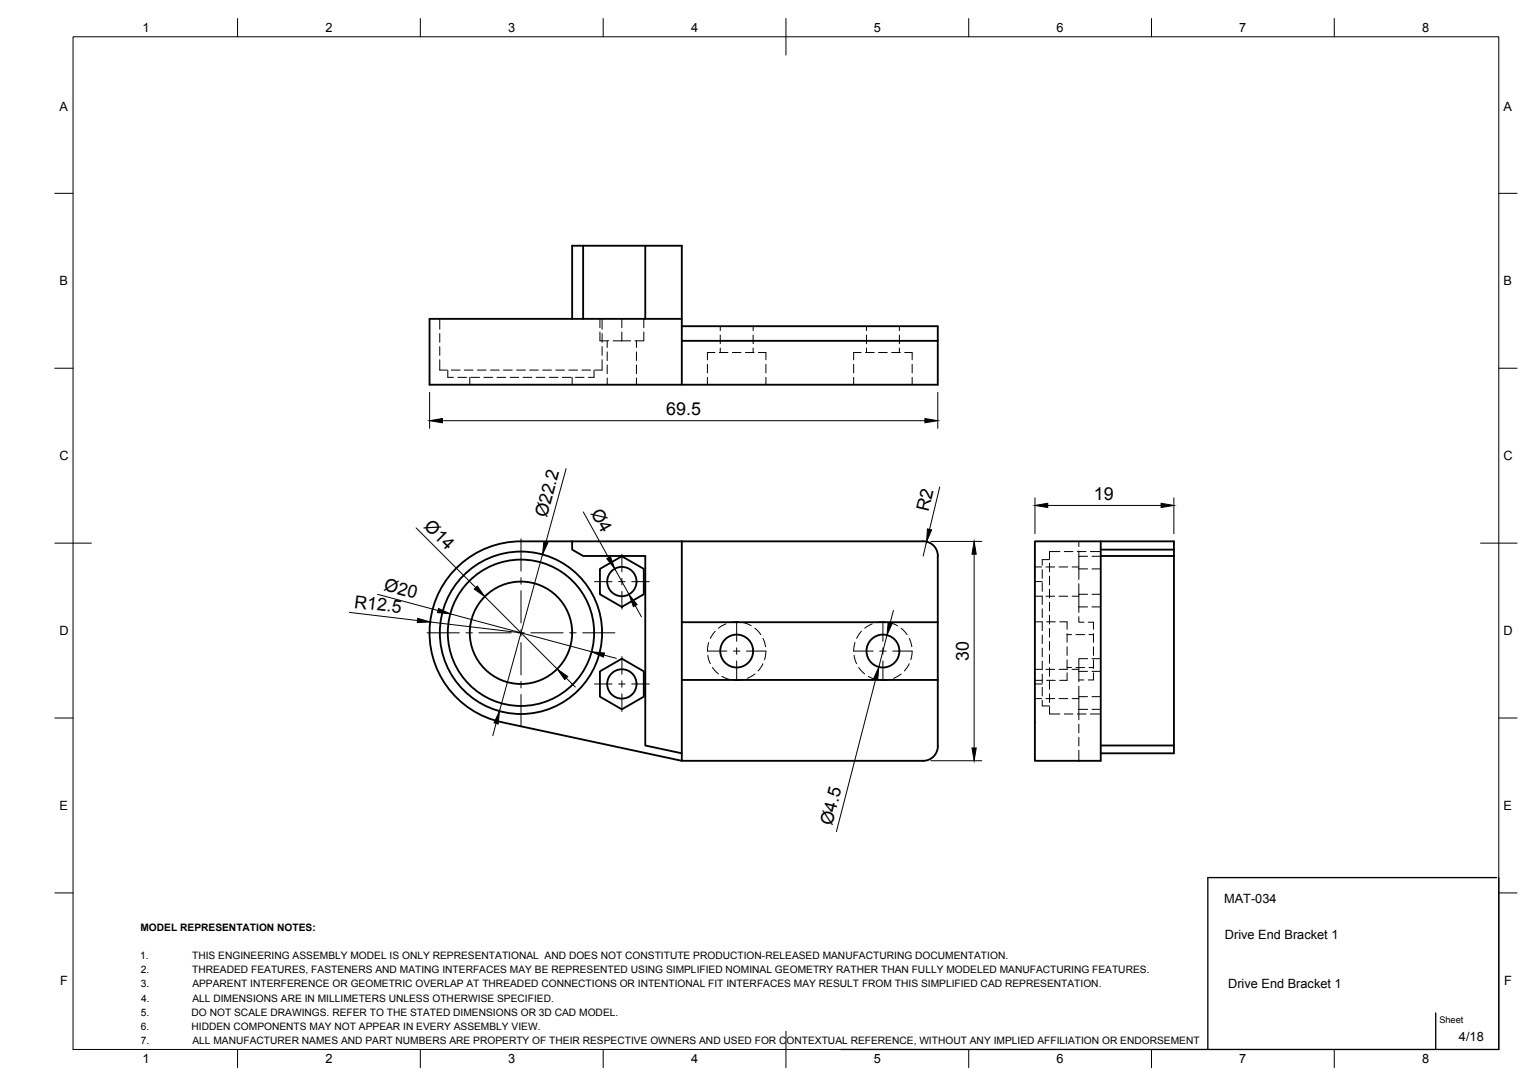
ISO-10303-21;
HEADER;
/* Generated by software containing ST-Developer
 * from STEP Tools, Inc. (www.steptools.com) 
 */

FILE_DESCRIPTION(
/* description */ ('STEP AP214'),
/* implementation_level */ '2;1');

FILE_NAME(
/* name */ 'Drive End Bracket 1.step',
/* time_stamp */ '2026-11-14T09:24:36-08:00',
/* author */ (''),
/* organization */ (''),
/* preprocessor_version */ 'ST-DEVELOPER v20.2',
/* originating_system */ 'Autodesk Translation Framework v15.17.0.0',
/* authorisation */ '');

FILE_SCHEMA (('AUTOMOTIVE_DESIGN { 1 0 10303 214 3 1 1 }'));
ENDSEC;

DATA;
#10=MECHANICAL_DESIGN_GEOMETRIC_PRESENTATION_REPRESENTATION('',(#203),#18867);
#171=SHAPE_REPRESENTATION_RELATIONSHIP('SRR','None',#18935,#187);
#187=ADVANCED_BREP_SHAPE_REPRESENTATION('',(#227),#18851);
#203=STYLED_ITEM('',(#19024),#227);
#227=MANIFOLD_SOLID_BREP('Body1',#10958);
#251=FACE_BOUND('',#1334,.T.);
#252=FACE_BOUND('',#1335,.T.);
#253=FACE_BOUND('',#1336,.T.);
#254=FACE_BOUND('',#1343,.T.);
#255=FACE_BOUND('',#1344,.T.);
#256=FACE_BOUND('',#1345,.T.);
#257=FACE_BOUND('',#1346,.T.);
#258=FACE_BOUND('',#1347,.T.);
#259=FACE_BOUND('',#1349,.T.);
#260=FACE_BOUND('',#1351,.T.);
#261=FACE_BOUND('',#1358,.T.);
#262=FACE_BOUND('',#1360,.T.);
#263=FACE_BOUND('',#1368,.T.);
#264=FACE_BOUND('',#1376,.T.);
#265=FACE_BOUND('',#1381,.T.);
#266=FACE_BOUND('',#1382,.T.);
#381=PLANE('',#11188);
#382=PLANE('',#11189);
#383=PLANE('',#11191);
#384=PLANE('',#11193);
#385=PLANE('',#11195);
#386=PLANE('',#11198);
#387=PLANE('',#11199);
#388=PLANE('',#11200);
#389=PLANE('',#11201);
#390=PLANE('',#11204);
#391=PLANE('',#11205);
#392=PLANE('',#11206);
#393=PLANE('',#11207);
#394=PLANE('',#11208);
#395=PLANE('',#11211);
#396=PLANE('',#11212);
#397=PLANE('',#11213);
#398=PLANE('',#11214);
#399=PLANE('',#11215);
#400=PLANE('',#11216);
#401=PLANE('',#11217);
#402=PLANE('',#11218);
#403=PLANE('',#11219);
#404=PLANE('',#11220);
#405=PLANE('',#11221);
#406=PLANE('',#11222);
#407=PLANE('',#11223);
#408=PLANE('',#11224);
#409=PLANE('',#11225);
#410=PLANE('',#11226);
#411=PLANE('',#11227);
#412=PLANE('',#11228);
#413=PLANE('',#11229);
#414=PLANE('',#11230);
#415=PLANE('',#11231);
#416=PLANE('',#11232);
#725=FACE_OUTER_BOUND('',#1321,.T.);
#726=FACE_OUTER_BOUND('',#1322,.T.);
#727=FACE_OUTER_BOUND('',#1323,.T.);
#728=FACE_OUTER_BOUND('',#1324,.T.);
#729=FACE_OUTER_BOUND('',#1325,.T.);
#730=FACE_OUTER_BOUND('',#1326,.T.);
#731=FACE_OUTER_BOUND('',#1327,.T.);
#732=FACE_OUTER_BOUND('',#1328,.T.);
#733=FACE_OUTER_BOUND('',#1329,.T.);
#734=FACE_OUTER_BOUND('',#1330,.T.);
#735=FACE_OUTER_BOUND('',#1331,.T.);
#736=FACE_OUTER_BOUND('',#1332,.T.);
#737=FACE_OUTER_BOUND('',#1333,.T.);
#738=FACE_OUTER_BOUND('',#1337,.T.);
#739=FACE_OUTER_BOUND('',#1338,.T.);
#740=FACE_OUTER_BOUND('',#1339,.T.);
#741=FACE_OUTER_BOUND('',#1340,.T.);
#742=FACE_OUTER_BOUND('',#1341,.T.);
#743=FACE_OUTER_BOUND('',#1342,.T.);
#744=FACE_OUTER_BOUND('',#1348,.T.);
#745=FACE_OUTER_BOUND('',#1350,.T.);
#746=FACE_OUTER_BOUND('',#1352,.T.);
#747=FACE_OUTER_BOUND('',#1353,.T.);
#748=FACE_OUTER_BOUND('',#1354,.T.);
#749=FACE_OUTER_BOUND('',#1355,.T.);
#750=FACE_OUTER_BOUND('',#1356,.T.);
#751=FACE_OUTER_BOUND('',#1357,.T.);
#752=FACE_OUTER_BOUND('',#1359,.T.);
#753=FACE_OUTER_BOUND('',#1361,.T.);
#754=FACE_OUTER_BOUND('',#1362,.T.);
#755=FACE_OUTER_BOUND('',#1363,.T.);
#756=FACE_OUTER_BOUND('',#1364,.T.);
#757=FACE_OUTER_BOUND('',#1365,.T.);
#758=FACE_OUTER_BOUND('',#1366,.T.);
#759=FACE_OUTER_BOUND('',#1367,.T.);
#760=FACE_OUTER_BOUND('',#1369,.T.);
#761=FACE_OUTER_BOUND('',#1370,.T.);
#762=FACE_OUTER_BOUND('',#1371,.T.);
#763=FACE_OUTER_BOUND('',#1372,.T.);
#764=FACE_OUTER_BOUND('',#1373,.T.);
#765=FACE_OUTER_BOUND('',#1374,.T.);
#766=FACE_OUTER_BOUND('',#1375,.T.);
#767=FACE_OUTER_BOUND('',#1377,.T.);
#768=FACE_OUTER_BOUND('',#1378,.T.);
#769=FACE_OUTER_BOUND('',#1379,.T.);
#770=FACE_OUTER_BOUND('',#1380,.T.);
#771=FACE_OUTER_BOUND('',#1383,.T.);
#772=FACE_OUTER_BOUND('',#1384,.T.);
#1321=EDGE_LOOP('',(#7108,#7109,#7110,#7111));
#1322=EDGE_LOOP('',(#7112,#7113,#7114,#7115));
#1323=EDGE_LOOP('',(#7116,#7117,#7118,#7119));
#1324=EDGE_LOOP('',(#7120,#7121,#7122,#7123));
#1325=EDGE_LOOP('',(#7124,#7125,#7126,#7127));
#1326=EDGE_LOOP('',(#7128,#7129,#7130,#7131));
#1327=EDGE_LOOP('',(#7132,#7133,#7134,#7135));
#1328=EDGE_LOOP('',(#7136,#7137,#7138,#7139));
#1329=EDGE_LOOP('',(#7140,#7141,#7142,#7143));
#1330=EDGE_LOOP('',(#7144,#7145,#7146,#7147,#7148,#7149,#7150,#7151,#7152,
#7153));
#1331=EDGE_LOOP('',(#7154,#7155,#7156,#7157,#7158));
#1332=EDGE_LOOP('',(#7159,#7160,#7161,#7162,#7163));
#1333=EDGE_LOOP('',(#7164,#7165,#7166,#7167,#7168,#7169,#7170,#7171,#7172));
#1334=EDGE_LOOP('',(#7173,#7174,#7175,#7176,#7177,#7178));
#1335=EDGE_LOOP('',(#7179,#7180,#7181,#7182,#7183,#7184));
#1336=EDGE_LOOP('',(#7185));
#1337=EDGE_LOOP('',(#7186,#7187,#7188,#7189,#7190));
#1338=EDGE_LOOP('',(#7191,#7192,#7193,#7194));
#1339=EDGE_LOOP('',(#7195,#7196,#7197,#7198,#7199,#7200,#7201,#7202));
#1340=EDGE_LOOP('',(#7203,#7204,#7205,#7206,#7207,#7208,#7209,#7210));
#1341=EDGE_LOOP('',(#7211,#7212,#7213,#7214));
#1342=EDGE_LOOP('',(#7215,#7216,#7217,#7218,#7219,#7220,#7221));
#1343=EDGE_LOOP('',(#7222));
#1344=EDGE_LOOP('',(#7223));
#1345=EDGE_LOOP('',(#7224));
#1346=EDGE_LOOP('',(#7225));
#1347=EDGE_LOOP('',(#7226));
#1348=EDGE_LOOP('',(#7227));
#1349=EDGE_LOOP('',(#7228));
#1350=EDGE_LOOP('',(#7229));
#1351=EDGE_LOOP('',(#7230));
#1352=EDGE_LOOP('',(#7231,#7232,#7233,#7234));
#1353=EDGE_LOOP('',(#7235,#7236,#7237,#7238));
#1354=EDGE_LOOP('',(#7239,#7240,#7241,#7242,#7243,#7244,#7245));
#1355=EDGE_LOOP('',(#7246,#7247,#7248,#7249));
#1356=EDGE_LOOP('',(#7250,#7251,#7252,#7253));
#1357=EDGE_LOOP('',(#7254));
#1358=EDGE_LOOP('',(#7255));
#1359=EDGE_LOOP('',(#7256));
#1360=EDGE_LOOP('',(#7257));
#1361=EDGE_LOOP('',(#7258,#7259,#7260,#7261));
#1362=EDGE_LOOP('',(#7262,#7263,#7264,#7265));
#1363=EDGE_LOOP('',(#7266,#7267,#7268,#7269));
#1364=EDGE_LOOP('',(#7270,#7271,#7272,#7273));
#1365=EDGE_LOOP('',(#7274,#7275,#7276,#7277));
#1366=EDGE_LOOP('',(#7278,#7279,#7280,#7281));
#1367=EDGE_LOOP('',(#7282,#7283,#7284,#7285,#7286,#7287));
#1368=EDGE_LOOP('',(#7288));
#1369=EDGE_LOOP('',(#7289,#7290,#7291,#7292));
#1370=EDGE_LOOP('',(#7293,#7294,#7295,#7296));
#1371=EDGE_LOOP('',(#7297,#7298,#7299,#7300));
#1372=EDGE_LOOP('',(#7301,#7302,#7303,#7304));
#1373=EDGE_LOOP('',(#7305,#7306,#7307,#7308));
#1374=EDGE_LOOP('',(#7309,#7310,#7311,#7312));
#1375=EDGE_LOOP('',(#7313,#7314,#7315,#7316,#7317,#7318));
#1376=EDGE_LOOP('',(#7319));
#1377=EDGE_LOOP('',(#7320,#7321,#7322,#7323));
#1378=EDGE_LOOP('',(#7324,#7325,#7326,#7327));
#1379=EDGE_LOOP('',(#7328,#7329,#7330,#7331));
#1380=EDGE_LOOP('',(#7332,#7333,#7334,#7335));
#1381=EDGE_LOOP('',(#7336));
#1382=EDGE_LOOP('',(#7337));
#1383=EDGE_LOOP('',(#7338,#7339,#7340,#7341));
#1384=EDGE_LOOP('',(#7342,#7343,#7344,#7345));
#2047=LINE('',#15611,#3061);
#2048=LINE('',#15617,#3062);
#2049=LINE('',#15623,#3063);
#2050=LINE('',#15629,#3064);
#2051=LINE('',#15635,#3065);
#2052=LINE('',#15641,#3066);
#2053=LINE('',#15647,#3067);
#2054=LINE('',#15653,#3068);
#2055=LINE('',#15659,#3069);
#2056=LINE('',#15664,#3070);
#2057=LINE('',#15666,#3071);
#2058=LINE('',#15668,#3072);
#2059=LINE('',#15670,#3073);
#2060=LINE('',#15672,#3074);
#2061=LINE('',#15674,#3075);
#2062=LINE('',#15676,#3076);
#2063=LINE('',#15678,#3077);
#2064=LINE('',#15680,#3078);
#2065=LINE('',#15681,#3079);
#2066=LINE('',#15684,#3080);
#2067=LINE('',#15686,#3081);
#2068=LINE('',#15689,#3082);
#2069=LINE('',#15692,#3083);
#2070=LINE('',#15694,#3084);
#2071=LINE('',#15697,#3085);
#2072=LINE('',#15701,#3086);
#2073=LINE('',#15703,#3087);
#2074=LINE('',#15705,#3088);
#2075=LINE('',#15707,#3089);
#2076=LINE('',#15710,#3090);
#2077=LINE('',#15712,#3091);
#2078=LINE('',#15713,#3092);
#2079=LINE('',#15716,#3093);
#2080=LINE('',#15718,#3094);
#2081=LINE('',#15720,#3095);
#2082=LINE('',#15722,#3096);
#2083=LINE('',#15724,#3097);
#2084=LINE('',#15725,#3098);
#2085=LINE('',#15728,#3099);
#2086=LINE('',#15730,#3100);
#2087=LINE('',#15732,#3101);
#2088=LINE('',#15734,#3102);
#2089=LINE('',#15736,#3103);
#2090=LINE('',#15737,#3104);
#2091=LINE('',#15740,#3105);
#2092=LINE('',#15742,#3106);
#2093=LINE('',#15743,#3107);
#2094=LINE('',#15746,#3108);
#2095=LINE('',#15750,#3109);
#2096=LINE('',#15751,#3110);
#2097=LINE('',#15753,#3111);
#2098=LINE('',#15754,#3112);
#2099=LINE('',#15757,#3113);
#2100=LINE('',#15759,#3114);
#2101=LINE('',#15761,#3115);
#2102=LINE('',#15762,#3116);
#2103=LINE('',#15764,#3117);
#2104=LINE('',#15765,#3118);
#2105=LINE('',#15768,#3119);
#2106=LINE('',#15769,#3120);
#2107=LINE('',#15777,#3121);
#2108=LINE('',#15778,#3122);
#2109=LINE('',#15781,#3123);
#2110=LINE('',#15782,#3124);
#2111=LINE('',#15785,#3125);
#2112=LINE('',#15787,#3126);
#2113=LINE('',#15788,#3127);
#2114=LINE('',#15795,#3128);
#2115=LINE('',#15797,#3129);
#2116=LINE('',#15798,#3130);
#2117=LINE('',#15801,#3131);
#2118=LINE('',#15802,#3132);
#2119=LINE('',#15805,#3133);
#2120=LINE('',#15806,#3134);
#2121=LINE('',#15809,#3135);
#2122=LINE('',#15810,#3136);
#2123=LINE('',#15813,#3137);
#2124=LINE('',#15814,#3138);
#2125=LINE('',#15816,#3139);
#2126=LINE('',#15820,#3140);
#2127=LINE('',#15822,#3141);
#2128=LINE('',#15823,#3142);
#2129=LINE('',#15826,#3143);
#2130=LINE('',#15827,#3144);
#2131=LINE('',#15830,#3145);
#2132=LINE('',#15831,#3146);
#2133=LINE('',#15834,#3147);
#2134=LINE('',#15835,#3148);
#2135=LINE('',#15838,#3149);
#2136=LINE('',#15839,#3150);
#2137=LINE('',#15841,#3151);
#2138=LINE('',#15844,#3152);
#2139=LINE('',#15846,#3153);
#2140=LINE('',#15849,#3154);
#2141=LINE('',#15850,#3155);
#3061=VECTOR('',#12311,2.);
#3062=VECTOR('',#12318,2.);
#3063=VECTOR('',#12325,4.);
#3064=VECTOR('',#12332,2.25);
#3065=VECTOR('',#12339,4.);
#3066=VECTOR('',#12346,2.25);
#3067=VECTOR('',#12353,7.00000000000001);
#3068=VECTOR('',#12360,10.);
#3069=VECTOR('',#12367,11.1);
#3070=VECTOR('',#12372,1000.);
#3071=VECTOR('',#12373,1000.);
#3072=VECTOR('',#12374,1000.);
#3073=VECTOR('',#12375,1000.);
#3074=VECTOR('',#12376,1000.);
#3075=VECTOR('',#12377,1000.);
#3076=VECTOR('',#12378,1000.);
#3077=VECTOR('',#12379,1000.);
#3078=VECTOR('',#12380,1000.);
#3079=VECTOR('',#12381,1000.);
#3080=VECTOR('',#12384,1000.);
#3081=VECTOR('',#12385,1000.);
#3082=VECTOR('',#12388,1000.);
#3083=VECTOR('',#12391,1000.);
#3084=VECTOR('',#12392,1000.);
#3085=VECTOR('',#12395,1000.);
#3086=VECTOR('',#12398,1000.);
#3087=VECTOR('',#12399,1000.);
#3088=VECTOR('',#12400,1000.);
#3089=VECTOR('',#12401,1000.);
#3090=VECTOR('',#12404,1000.);
#3091=VECTOR('',#12405,1000.);
#3092=VECTOR('',#12406,1000.);
#3093=VECTOR('',#12407,1000.);
#3094=VECTOR('',#12408,1000.);
#3095=VECTOR('',#12409,1000.);
#3096=VECTOR('',#12410,1000.);
#3097=VECTOR('',#12411,1000.);
#3098=VECTOR('',#12412,1000.);
#3099=VECTOR('',#12413,1000.);
#3100=VECTOR('',#12414,1000.);
#3101=VECTOR('',#12415,1000.);
#3102=VECTOR('',#12416,1000.);
#3103=VECTOR('',#12417,1000.);
#3104=VECTOR('',#12418,1000.);
#3105=VECTOR('',#12421,1000.);
#3106=VECTOR('',#12422,1000.);
#3107=VECTOR('',#12423,1000.);
#3108=VECTOR('',#12426,1000.);
#3109=VECTOR('',#12431,1000.);
#3110=VECTOR('',#12432,1000.);
#3111=VECTOR('',#12433,1000.);
#3112=VECTOR('',#12434,1000.);
#3113=VECTOR('',#12437,1000.);
#3114=VECTOR('',#12438,1000.);
#3115=VECTOR('',#12439,1000.);
#3116=VECTOR('',#12440,1000.);
#3117=VECTOR('',#12441,1000.);
#3118=VECTOR('',#12442,1000.);
#3119=VECTOR('',#12445,1000.);
#3120=VECTOR('',#12446,1000.);
#3121=VECTOR('',#12459,1000.);
#3122=VECTOR('',#12460,1000.);
#3123=VECTOR('',#12463,1000.);
#3124=VECTOR('',#12464,1000.);
#3125=VECTOR('',#12467,1000.);
#3126=VECTOR('',#12468,1000.);
#3127=VECTOR('',#12469,1000.);
#3128=VECTOR('',#12480,1000.);
#3129=VECTOR('',#12481,1000.);
#3130=VECTOR('',#12482,1000.);
#3131=VECTOR('',#12485,1000.);
#3132=VECTOR('',#12486,1000.);
#3133=VECTOR('',#12489,1000.);
#3134=VECTOR('',#12490,1000.);
#3135=VECTOR('',#12493,1000.);
#3136=VECTOR('',#12494,1000.);
#3137=VECTOR('',#12497,1000.);
#3138=VECTOR('',#12498,1000.);
#3139=VECTOR('',#12501,1000.);
#3140=VECTOR('',#12506,1000.);
#3141=VECTOR('',#12507,1000.);
#3142=VECTOR('',#12508,1000.);
#3143=VECTOR('',#12511,1000.);
#3144=VECTOR('',#12512,1000.);
#3145=VECTOR('',#12515,1000.);
#3146=VECTOR('',#12516,1000.);
#3147=VECTOR('',#12519,1000.);
#3148=VECTOR('',#12520,1000.);
#3149=VECTOR('',#12523,1000.);
#3150=VECTOR('',#12524,1000.);
#3151=VECTOR('',#12527,1000.);
#3152=VECTOR('',#12532,1000.);
#3153=VECTOR('',#12535,1000.);
#3154=VECTOR('',#12540,1000.);
#3155=VECTOR('',#12541,1000.);
#4075=CIRCLE('',#11162,2.);
#4076=CIRCLE('',#11163,2.);
#4077=CIRCLE('',#11165,2.);
#4078=CIRCLE('',#11166,2.);
#4079=CIRCLE('',#11168,4.);
#4080=CIRCLE('',#11169,4.);
#4081=CIRCLE('',#11171,2.25000000000001);
#4082=CIRCLE('',#11172,2.25);
#4083=CIRCLE('',#11174,4.);
#4084=CIRCLE('',#11175,4.);
#4085=CIRCLE('',#11177,2.25000000000001);
#4086=CIRCLE('',#11178,2.25);
#4087=CIRCLE('',#11180,7.00000000000001);
#4088=CIRCLE('',#11181,7.00000000000001);
#4089=CIRCLE('',#11183,10.);
#4090=CIRCLE('',#11184,10.);
#4091=CIRCLE('',#11186,11.1);
#4092=CIRCLE('',#11187,11.1);
#4093=CIRCLE('',#11190,2.);
#4094=CIRCLE('',#11192,2.);
#4095=CIRCLE('',#11194,12.5);
#4096=CIRCLE('',#11197,12.5);
#4097=CIRCLE('',#11202,2.);
#4098=CIRCLE('',#11203,2.);
#4574=VERTEX_POINT('',#15608);
#4575=VERTEX_POINT('',#15610);
#4576=VERTEX_POINT('',#15614);
#4577=VERTEX_POINT('',#15616);
#4578=VERTEX_POINT('',#15620);
#4579=VERTEX_POINT('',#15622);
#4580=VERTEX_POINT('',#15626);
#4581=VERTEX_POINT('',#15628);
#4582=VERTEX_POINT('',#15632);
#4583=VERTEX_POINT('',#15634);
#4584=VERTEX_POINT('',#15638);
#4585=VERTEX_POINT('',#15640);
#4586=VERTEX_POINT('',#15644);
#4587=VERTEX_POINT('',#15646);
#4588=VERTEX_POINT('',#15650);
#4589=VERTEX_POINT('',#15652);
#4590=VERTEX_POINT('',#15656);
#4591=VERTEX_POINT('',#15658);
#4592=VERTEX_POINT('',#15662);
#4593=VERTEX_POINT('',#15663);
#4594=VERTEX_POINT('',#15665);
#4595=VERTEX_POINT('',#15667);
#4596=VERTEX_POINT('',#15669);
#4597=VERTEX_POINT('',#15671);
#4598=VERTEX_POINT('',#15673);
#4599=VERTEX_POINT('',#15675);
#4600=VERTEX_POINT('',#15677);
#4601=VERTEX_POINT('',#15679);
#4602=VERTEX_POINT('',#15683);
#4603=VERTEX_POINT('',#15685);
#4604=VERTEX_POINT('',#15687);
#4605=VERTEX_POINT('',#15691);
#4606=VERTEX_POINT('',#15693);
#4607=VERTEX_POINT('',#15695);
#4608=VERTEX_POINT('',#15699);
#4609=VERTEX_POINT('',#15700);
#4610=VERTEX_POINT('',#15702);
#4611=VERTEX_POINT('',#15704);
#4612=VERTEX_POINT('',#15706);
#4613=VERTEX_POINT('',#15708);
#4614=VERTEX_POINT('',#15711);
#4615=VERTEX_POINT('',#15714);
#4616=VERTEX_POINT('',#15715);
#4617=VERTEX_POINT('',#15717);
#4618=VERTEX_POINT('',#15719);
#4619=VERTEX_POINT('',#15721);
#4620=VERTEX_POINT('',#15723);
#4621=VERTEX_POINT('',#15726);
#4622=VERTEX_POINT('',#15727);
#4623=VERTEX_POINT('',#15729);
#4624=VERTEX_POINT('',#15731);
#4625=VERTEX_POINT('',#15733);
#4626=VERTEX_POINT('',#15735);
#4627=VERTEX_POINT('',#15739);
#4628=VERTEX_POINT('',#15741);
#4629=VERTEX_POINT('',#15745);
#4630=VERTEX_POINT('',#15749);
#4631=VERTEX_POINT('',#15752);
#4632=VERTEX_POINT('',#15756);
#4633=VERTEX_POINT('',#15758);
#4634=VERTEX_POINT('',#15760);
#4635=VERTEX_POINT('',#15763);
#4636=VERTEX_POINT('',#15767);
#4637=VERTEX_POINT('',#15776);
#4638=VERTEX_POINT('',#15780);
#4639=VERTEX_POINT('',#15784);
#4640=VERTEX_POINT('',#15786);
#4641=VERTEX_POINT('',#15794);
#4642=VERTEX_POINT('',#15796);
#4643=VERTEX_POINT('',#15800);
#4644=VERTEX_POINT('',#15804);
#4645=VERTEX_POINT('',#15808);
#4646=VERTEX_POINT('',#15812);
#4647=VERTEX_POINT('',#15819);
#4648=VERTEX_POINT('',#15821);
#4649=VERTEX_POINT('',#15825);
#4650=VERTEX_POINT('',#15829);
#4651=VERTEX_POINT('',#15833);
#4652=VERTEX_POINT('',#15837);
#5587=EDGE_CURVE('',#4574,#4574,#4075,.T.);
#5588=EDGE_CURVE('',#4574,#4575,#2047,.T.);
#5589=EDGE_CURVE('',#4575,#4575,#4076,.T.);
#5590=EDGE_CURVE('',#4576,#4576,#4077,.T.);
#5591=EDGE_CURVE('',#4576,#4577,#2048,.T.);
#5592=EDGE_CURVE('',#4577,#4577,#4078,.T.);
#5593=EDGE_CURVE('',#4578,#4578,#4079,.T.);
#5594=EDGE_CURVE('',#4578,#4579,#2049,.T.);
#5595=EDGE_CURVE('',#4579,#4579,#4080,.T.);
#5596=EDGE_CURVE('',#4580,#4580,#4081,.T.);
#5597=EDGE_CURVE('',#4580,#4581,#2050,.T.);
#5598=EDGE_CURVE('',#4581,#4581,#4082,.T.);
#5599=EDGE_CURVE('',#4582,#4582,#4083,.T.);
#5600=EDGE_CURVE('',#4582,#4583,#2051,.T.);
#5601=EDGE_CURVE('',#4583,#4583,#4084,.T.);
#5602=EDGE_CURVE('',#4584,#4584,#4085,.T.);
#5603=EDGE_CURVE('',#4584,#4585,#2052,.T.);
#5604=EDGE_CURVE('',#4585,#4585,#4086,.T.);
#5605=EDGE_CURVE('',#4586,#4586,#4087,.T.);
#5606=EDGE_CURVE('',#4586,#4587,#2053,.T.);
#5607=EDGE_CURVE('',#4587,#4587,#4088,.T.);
#5608=EDGE_CURVE('',#4588,#4588,#4089,.T.);
#5609=EDGE_CURVE('',#4588,#4589,#2054,.T.);
#5610=EDGE_CURVE('',#4589,#4589,#4090,.T.);
#5611=EDGE_CURVE('',#4590,#4590,#4091,.T.);
#5612=EDGE_CURVE('',#4590,#4591,#2055,.T.);
#5613=EDGE_CURVE('',#4591,#4591,#4092,.T.);
#5614=EDGE_CURVE('',#4592,#4593,#2056,.T.);
#5615=EDGE_CURVE('',#4594,#4592,#2057,.T.);
#5616=EDGE_CURVE('',#4594,#4595,#2058,.T.);
#5617=EDGE_CURVE('',#4595,#4596,#2059,.T.);
#5618=EDGE_CURVE('',#4596,#4597,#2060,.T.);
#5619=EDGE_CURVE('',#4598,#4597,#2061,.T.);
#5620=EDGE_CURVE('',#4598,#4599,#2062,.T.);
#5621=EDGE_CURVE('',#4600,#4599,#2063,.T.);
#5622=EDGE_CURVE('',#4600,#4601,#2064,.T.);
#5623=EDGE_CURVE('',#4601,#4593,#2065,.T.);
#5624=EDGE_CURVE('',#4593,#4602,#2066,.T.);
#5625=EDGE_CURVE('',#4601,#4603,#2067,.T.);
#5626=EDGE_CURVE('',#4603,#4604,#4093,.T.);
#5627=EDGE_CURVE('',#4604,#4602,#2068,.T.);
#5628=EDGE_CURVE('',#4605,#4595,#2069,.T.);
#5629=EDGE_CURVE('',#4605,#4606,#2070,.T.);
#5630=EDGE_CURVE('',#4606,#4607,#4094,.T.);
#5631=EDGE_CURVE('',#4596,#4607,#2071,.T.);
#5632=EDGE_CURVE('',#4608,#4609,#2072,.T.);
#5633=EDGE_CURVE('',#4609,#4610,#2073,.T.);
#5634=EDGE_CURVE('',#4610,#4611,#2074,.T.);
#5635=EDGE_CURVE('',#4611,#4612,#2075,.T.);
#5636=EDGE_CURVE('',#4613,#4612,#4095,.T.);
#5637=EDGE_CURVE('',#4613,#4600,#2076,.T.);
#5638=EDGE_CURVE('',#4614,#4599,#2077,.T.);
#5639=EDGE_CURVE('',#4608,#4614,#2078,.T.);
#5640=EDGE_CURVE('',#4615,#4616,#2079,.T.);
#5641=EDGE_CURVE('',#4617,#4615,#2080,.T.);
#5642=EDGE_CURVE('',#4618,#4617,#2081,.T.);
#5643=EDGE_CURVE('',#4619,#4618,#2082,.T.);
#5644=EDGE_CURVE('',#4620,#4619,#2083,.T.);
#5645=EDGE_CURVE('',#4616,#4620,#2084,.T.);
#5646=EDGE_CURVE('',#4621,#4622,#2085,.T.);
#5647=EDGE_CURVE('',#4623,#4621,#2086,.T.);
#5648=EDGE_CURVE('',#4624,#4623,#2087,.T.);
#5649=EDGE_CURVE('',#4625,#4624,#2088,.T.);
#5650=EDGE_CURVE('',#4626,#4625,#2089,.T.);
#5651=EDGE_CURVE('',#4622,#4626,#2090,.T.);
#5652=EDGE_CURVE('',#4627,#4613,#2091,.T.);
#5653=EDGE_CURVE('',#4627,#4628,#2092,.T.);
#5654=EDGE_CURVE('',#4628,#4601,#2093,.T.);
#5655=EDGE_CURVE('',#4629,#4612,#2094,.T.);
#5656=EDGE_CURVE('',#4627,#4629,#4096,.T.);
#5657=EDGE_CURVE('',#4607,#4630,#2095,.T.);
#5658=EDGE_CURVE('',#4630,#4629,#2096,.T.);
#5659=EDGE_CURVE('',#4611,#4631,#2097,.T.);
#5660=EDGE_CURVE('',#4631,#4597,#2098,.T.);
#5661=EDGE_CURVE('',#4632,#4606,#2099,.T.);
#5662=EDGE_CURVE('',#4633,#4605,#2100,.T.);
#5663=EDGE_CURVE('',#4634,#4633,#2101,.T.);
#5664=EDGE_CURVE('',#4634,#4602,#2102,.T.);
#5665=EDGE_CURVE('',#4604,#4635,#2103,.T.);
#5666=EDGE_CURVE('',#4632,#4635,#2104,.T.);
#5667=EDGE_CURVE('',#4636,#4603,#2105,.T.);
#5668=EDGE_CURVE('',#4636,#4628,#2106,.T.);
#5669=EDGE_CURVE('',#4635,#4636,#4097,.T.);
#5670=EDGE_CURVE('',#4630,#4632,#4098,.T.);
#5671=EDGE_CURVE('',#4637,#4598,#2107,.T.);
#5672=EDGE_CURVE('',#4637,#4614,#2108,.T.);
#5673=EDGE_CURVE('',#4638,#4637,#2109,.T.);
#5674=EDGE_CURVE('',#4638,#4608,#2110,.T.);
#5675=EDGE_CURVE('',#4639,#4631,#2111,.T.);
#5676=EDGE_CURVE('',#4639,#4640,#2112,.T.);
#5677=EDGE_CURVE('',#4640,#4638,#2113,.T.);
#5678=EDGE_CURVE('',#4641,#4621,#2114,.T.);
#5679=EDGE_CURVE('',#4642,#4641,#2115,.T.);
#5680=EDGE_CURVE('',#4642,#4623,#2116,.T.);
#5681=EDGE_CURVE('',#4643,#4642,#2117,.T.);
#5682=EDGE_CURVE('',#4643,#4624,#2118,.T.);
#5683=EDGE_CURVE('',#4644,#4643,#2119,.T.);
#5684=EDGE_CURVE('',#4644,#4625,#2120,.T.);
#5685=EDGE_CURVE('',#4645,#4644,#2121,.T.);
#5686=EDGE_CURVE('',#4645,#4626,#2122,.T.);
#5687=EDGE_CURVE('',#4646,#4645,#2123,.T.);
#5688=EDGE_CURVE('',#4646,#4622,#2124,.T.);
#5689=EDGE_CURVE('',#4641,#4646,#2125,.T.);
#5690=EDGE_CURVE('',#4647,#4615,#2126,.T.);
#5691=EDGE_CURVE('',#4648,#4647,#2127,.T.);
#5692=EDGE_CURVE('',#4648,#4617,#2128,.T.);
#5693=EDGE_CURVE('',#4649,#4648,#2129,.T.);
#5694=EDGE_CURVE('',#4649,#4618,#2130,.T.);
#5695=EDGE_CURVE('',#4650,#4649,#2131,.T.);
#5696=EDGE_CURVE('',#4650,#4619,#2132,.T.);
#5697=EDGE_CURVE('',#4651,#4650,#2133,.T.);
#5698=EDGE_CURVE('',#4651,#4620,#2134,.T.);
#5699=EDGE_CURVE('',#4652,#4651,#2135,.T.);
#5700=EDGE_CURVE('',#4652,#4616,#2136,.T.);
#5701=EDGE_CURVE('',#4647,#4652,#2137,.T.);
#5702=EDGE_CURVE('',#4640,#4609,#2138,.T.);
#5703=EDGE_CURVE('',#4610,#4639,#2139,.T.);
#5704=EDGE_CURVE('',#4592,#4634,#2140,.T.);
#5705=EDGE_CURVE('',#4633,#4594,#2141,.T.);
#7108=ORIENTED_EDGE('',*,*,#5587,.F.);
#7109=ORIENTED_EDGE('',*,*,#5588,.T.);
#7110=ORIENTED_EDGE('',*,*,#5589,.T.);
#7111=ORIENTED_EDGE('',*,*,#5588,.F.);
#7112=ORIENTED_EDGE('',*,*,#5590,.F.);
#7113=ORIENTED_EDGE('',*,*,#5591,.T.);
#7114=ORIENTED_EDGE('',*,*,#5592,.T.);
#7115=ORIENTED_EDGE('',*,*,#5591,.F.);
#7116=ORIENTED_EDGE('',*,*,#5593,.F.);
#7117=ORIENTED_EDGE('',*,*,#5594,.T.);
#7118=ORIENTED_EDGE('',*,*,#5595,.T.);
#7119=ORIENTED_EDGE('',*,*,#5594,.F.);
#7120=ORIENTED_EDGE('',*,*,#5596,.T.);
#7121=ORIENTED_EDGE('',*,*,#5597,.T.);
#7122=ORIENTED_EDGE('',*,*,#5598,.T.);
#7123=ORIENTED_EDGE('',*,*,#5597,.F.);
#7124=ORIENTED_EDGE('',*,*,#5599,.F.);
#7125=ORIENTED_EDGE('',*,*,#5600,.T.);
#7126=ORIENTED_EDGE('',*,*,#5601,.T.);
#7127=ORIENTED_EDGE('',*,*,#5600,.F.);
#7128=ORIENTED_EDGE('',*,*,#5602,.T.);
#7129=ORIENTED_EDGE('',*,*,#5603,.T.);
#7130=ORIENTED_EDGE('',*,*,#5604,.T.);
#7131=ORIENTED_EDGE('',*,*,#5603,.F.);
#7132=ORIENTED_EDGE('',*,*,#5605,.F.);
#7133=ORIENTED_EDGE('',*,*,#5606,.T.);
#7134=ORIENTED_EDGE('',*,*,#5607,.T.);
#7135=ORIENTED_EDGE('',*,*,#5606,.F.);
#7136=ORIENTED_EDGE('',*,*,#5608,.F.);
#7137=ORIENTED_EDGE('',*,*,#5609,.T.);
#7138=ORIENTED_EDGE('',*,*,#5610,.T.);
#7139=ORIENTED_EDGE('',*,*,#5609,.F.);
#7140=ORIENTED_EDGE('',*,*,#5611,.F.);
#7141=ORIENTED_EDGE('',*,*,#5612,.T.);
#7142=ORIENTED_EDGE('',*,*,#5613,.T.);
#7143=ORIENTED_EDGE('',*,*,#5612,.F.);
#7144=ORIENTED_EDGE('',*,*,#5614,.F.);
#7145=ORIENTED_EDGE('',*,*,#5615,.F.);
#7146=ORIENTED_EDGE('',*,*,#5616,.T.);
#7147=ORIENTED_EDGE('',*,*,#5617,.T.);
#7148=ORIENTED_EDGE('',*,*,#5618,.T.);
#7149=ORIENTED_EDGE('',*,*,#5619,.F.);
#7150=ORIENTED_EDGE('',*,*,#5620,.T.);
#7151=ORIENTED_EDGE('',*,*,#5621,.F.);
#7152=ORIENTED_EDGE('',*,*,#5622,.T.);
#7153=ORIENTED_EDGE('',*,*,#5623,.T.);
#7154=ORIENTED_EDGE('',*,*,#5624,.F.);
#7155=ORIENTED_EDGE('',*,*,#5623,.F.);
#7156=ORIENTED_EDGE('',*,*,#5625,.T.);
#7157=ORIENTED_EDGE('',*,*,#5626,.T.);
#7158=ORIENTED_EDGE('',*,*,#5627,.T.);
#7159=ORIENTED_EDGE('',*,*,#5628,.F.);
#7160=ORIENTED_EDGE('',*,*,#5629,.T.);
#7161=ORIENTED_EDGE('',*,*,#5630,.T.);
#7162=ORIENTED_EDGE('',*,*,#5631,.F.);
#7163=ORIENTED_EDGE('',*,*,#5617,.F.);
#7164=ORIENTED_EDGE('',*,*,#5632,.T.);
#7165=ORIENTED_EDGE('',*,*,#5633,.T.);
#7166=ORIENTED_EDGE('',*,*,#5634,.T.);
#7167=ORIENTED_EDGE('',*,*,#5635,.T.);
#7168=ORIENTED_EDGE('',*,*,#5636,.F.);
#7169=ORIENTED_EDGE('',*,*,#5637,.T.);
#7170=ORIENTED_EDGE('',*,*,#5621,.T.);
#7171=ORIENTED_EDGE('',*,*,#5638,.F.);
#7172=ORIENTED_EDGE('',*,*,#5639,.F.);
#7173=ORIENTED_EDGE('',*,*,#5640,.F.);
#7174=ORIENTED_EDGE('',*,*,#5641,.F.);
#7175=ORIENTED_EDGE('',*,*,#5642,.F.);
#7176=ORIENTED_EDGE('',*,*,#5643,.F.);
#7177=ORIENTED_EDGE('',*,*,#5644,.F.);
#7178=ORIENTED_EDGE('',*,*,#5645,.F.);
#7179=ORIENTED_EDGE('',*,*,#5646,.F.);
#7180=ORIENTED_EDGE('',*,*,#5647,.F.);
#7181=ORIENTED_EDGE('',*,*,#5648,.F.);
#7182=ORIENTED_EDGE('',*,*,#5649,.F.);
#7183=ORIENTED_EDGE('',*,*,#5650,.F.);
#7184=ORIENTED_EDGE('',*,*,#5651,.F.);
#7185=ORIENTED_EDGE('',*,*,#5613,.F.);
#7186=ORIENTED_EDGE('',*,*,#5637,.F.);
#7187=ORIENTED_EDGE('',*,*,#5652,.F.);
#7188=ORIENTED_EDGE('',*,*,#5653,.T.);
#7189=ORIENTED_EDGE('',*,*,#5654,.T.);
#7190=ORIENTED_EDGE('',*,*,#5622,.F.);
#7191=ORIENTED_EDGE('',*,*,#5636,.T.);
#7192=ORIENTED_EDGE('',*,*,#5655,.F.);
#7193=ORIENTED_EDGE('',*,*,#5656,.F.);
#7194=ORIENTED_EDGE('',*,*,#5652,.T.);
#7195=ORIENTED_EDGE('',*,*,#5631,.T.);
#7196=ORIENTED_EDGE('',*,*,#5657,.T.);
#7197=ORIENTED_EDGE('',*,*,#5658,.T.);
#7198=ORIENTED_EDGE('',*,*,#5655,.T.);
#7199=ORIENTED_EDGE('',*,*,#5635,.F.);
#7200=ORIENTED_EDGE('',*,*,#5659,.T.);
#7201=ORIENTED_EDGE('',*,*,#5660,.T.);
#7202=ORIENTED_EDGE('',*,*,#5618,.F.);
#7203=ORIENTED_EDGE('',*,*,#5661,.T.);
#7204=ORIENTED_EDGE('',*,*,#5629,.F.);
#7205=ORIENTED_EDGE('',*,*,#5662,.F.);
#7206=ORIENTED_EDGE('',*,*,#5663,.F.);
#7207=ORIENTED_EDGE('',*,*,#5664,.T.);
#7208=ORIENTED_EDGE('',*,*,#5627,.F.);
#7209=ORIENTED_EDGE('',*,*,#5665,.T.);
#7210=ORIENTED_EDGE('',*,*,#5666,.F.);
#7211=ORIENTED_EDGE('',*,*,#5667,.T.);
#7212=ORIENTED_EDGE('',*,*,#5625,.F.);
#7213=ORIENTED_EDGE('',*,*,#5654,.F.);
#7214=ORIENTED_EDGE('',*,*,#5668,.F.);
#7215=ORIENTED_EDGE('',*,*,#5666,.T.);
#7216=ORIENTED_EDGE('',*,*,#5669,.T.);
#7217=ORIENTED_EDGE('',*,*,#5668,.T.);
#7218=ORIENTED_EDGE('',*,*,#5653,.F.);
#7219=ORIENTED_EDGE('',*,*,#5656,.T.);
#7220=ORIENTED_EDGE('',*,*,#5658,.F.);
#7221=ORIENTED_EDGE('',*,*,#5670,.T.);
#7222=ORIENTED_EDGE('',*,*,#5587,.T.);
#7223=ORIENTED_EDGE('',*,*,#5590,.T.);
#7224=ORIENTED_EDGE('',*,*,#5595,.F.);
#7225=ORIENTED_EDGE('',*,*,#5601,.F.);
#7226=ORIENTED_EDGE('',*,*,#5605,.T.);
#7227=ORIENTED_EDGE('',*,*,#5611,.T.);
#7228=ORIENTED_EDGE('',*,*,#5610,.F.);
#7229=ORIENTED_EDGE('',*,*,#5608,.T.);
#7230=ORIENTED_EDGE('',*,*,#5607,.F.);
#7231=ORIENTED_EDGE('',*,*,#5638,.T.);
#7232=ORIENTED_EDGE('',*,*,#5620,.F.);
#7233=ORIENTED_EDGE('',*,*,#5671,.F.);
#7234=ORIENTED_EDGE('',*,*,#5672,.T.);
#7235=ORIENTED_EDGE('',*,*,#5673,.F.);
#7236=ORIENTED_EDGE('',*,*,#5674,.T.);
#7237=ORIENTED_EDGE('',*,*,#5639,.T.);
#7238=ORIENTED_EDGE('',*,*,#5672,.F.);
#7239=ORIENTED_EDGE('',*,*,#5675,.F.);
#7240=ORIENTED_EDGE('',*,*,#5676,.T.);
#7241=ORIENTED_EDGE('',*,*,#5677,.T.);
#7242=ORIENTED_EDGE('',*,*,#5673,.T.);
#7243=ORIENTED_EDGE('',*,*,#5671,.T.);
#7244=ORIENTED_EDGE('',*,*,#5619,.T.);
#7245=ORIENTED_EDGE('',*,*,#5660,.F.);
#7246=ORIENTED_EDGE('',*,*,#5626,.F.);
#7247=ORIENTED_EDGE('',*,*,#5667,.F.);
#7248=ORIENTED_EDGE('',*,*,#5669,.F.);
#7249=ORIENTED_EDGE('',*,*,#5665,.F.);
#7250=ORIENTED_EDGE('',*,*,#5630,.F.);
#7251=ORIENTED_EDGE('',*,*,#5661,.F.);
#7252=ORIENTED_EDGE('',*,*,#5670,.F.);
#7253=ORIENTED_EDGE('',*,*,#5657,.F.);
#7254=ORIENTED_EDGE('',*,*,#5599,.T.);
#7255=ORIENTED_EDGE('',*,*,#5604,.F.);
#7256=ORIENTED_EDGE('',*,*,#5593,.T.);
#7257=ORIENTED_EDGE('',*,*,#5598,.F.);
#7258=ORIENTED_EDGE('',*,*,#5647,.T.);
#7259=ORIENTED_EDGE('',*,*,#5678,.F.);
#7260=ORIENTED_EDGE('',*,*,#5679,.F.);
#7261=ORIENTED_EDGE('',*,*,#5680,.T.);
#7262=ORIENTED_EDGE('',*,*,#5648,.T.);
#7263=ORIENTED_EDGE('',*,*,#5680,.F.);
#7264=ORIENTED_EDGE('',*,*,#5681,.F.);
#7265=ORIENTED_EDGE('',*,*,#5682,.T.);
#7266=ORIENTED_EDGE('',*,*,#5649,.T.);
#7267=ORIENTED_EDGE('',*,*,#5682,.F.);
#7268=ORIENTED_EDGE('',*,*,#5683,.F.);
#7269=ORIENTED_EDGE('',*,*,#5684,.T.);
#7270=ORIENTED_EDGE('',*,*,#5650,.T.);
#7271=ORIENTED_EDGE('',*,*,#5684,.F.);
#7272=ORIENTED_EDGE('',*,*,#5685,.F.);
#7273=ORIENTED_EDGE('',*,*,#5686,.T.);
#7274=ORIENTED_EDGE('',*,*,#5651,.T.);
#7275=ORIENTED_EDGE('',*,*,#5686,.F.);
#7276=ORIENTED_EDGE('',*,*,#5687,.F.);
#7277=ORIENTED_EDGE('',*,*,#5688,.T.);
#7278=ORIENTED_EDGE('',*,*,#5646,.T.);
#7279=ORIENTED_EDGE('',*,*,#5688,.F.);
#7280=ORIENTED_EDGE('',*,*,#5689,.F.);
#7281=ORIENTED_EDGE('',*,*,#5678,.T.);
#7282=ORIENTED_EDGE('',*,*,#5679,.T.);
#7283=ORIENTED_EDGE('',*,*,#5689,.T.);
#7284=ORIENTED_EDGE('',*,*,#5687,.T.);
#7285=ORIENTED_EDGE('',*,*,#5685,.T.);
#7286=ORIENTED_EDGE('',*,*,#5683,.T.);
#7287=ORIENTED_EDGE('',*,*,#5681,.T.);
#7288=ORIENTED_EDGE('',*,*,#5592,.F.);
#7289=ORIENTED_EDGE('',*,*,#5641,.T.);
#7290=ORIENTED_EDGE('',*,*,#5690,.F.);
#7291=ORIENTED_EDGE('',*,*,#5691,.F.);
#7292=ORIENTED_EDGE('',*,*,#5692,.T.);
#7293=ORIENTED_EDGE('',*,*,#5642,.T.);
#7294=ORIENTED_EDGE('',*,*,#5692,.F.);
#7295=ORIENTED_EDGE('',*,*,#5693,.F.);
#7296=ORIENTED_EDGE('',*,*,#5694,.T.);
#7297=ORIENTED_EDGE('',*,*,#5643,.T.);
#7298=ORIENTED_EDGE('',*,*,#5694,.F.);
#7299=ORIENTED_EDGE('',*,*,#5695,.F.);
#7300=ORIENTED_EDGE('',*,*,#5696,.T.);
#7301=ORIENTED_EDGE('',*,*,#5644,.T.);
#7302=ORIENTED_EDGE('',*,*,#5696,.F.);
#7303=ORIENTED_EDGE('',*,*,#5697,.F.);
#7304=ORIENTED_EDGE('',*,*,#5698,.T.);
#7305=ORIENTED_EDGE('',*,*,#5645,.T.);
#7306=ORIENTED_EDGE('',*,*,#5698,.F.);
#7307=ORIENTED_EDGE('',*,*,#5699,.F.);
#7308=ORIENTED_EDGE('',*,*,#5700,.T.);
#7309=ORIENTED_EDGE('',*,*,#5640,.T.);
#7310=ORIENTED_EDGE('',*,*,#5700,.F.);
#7311=ORIENTED_EDGE('',*,*,#5701,.F.);
#7312=ORIENTED_EDGE('',*,*,#5690,.T.);
#7313=ORIENTED_EDGE('',*,*,#5691,.T.);
#7314=ORIENTED_EDGE('',*,*,#5701,.T.);
#7315=ORIENTED_EDGE('',*,*,#5699,.T.);
#7316=ORIENTED_EDGE('',*,*,#5697,.T.);
#7317=ORIENTED_EDGE('',*,*,#5695,.T.);
#7318=ORIENTED_EDGE('',*,*,#5693,.T.);
#7319=ORIENTED_EDGE('',*,*,#5589,.F.);
#7320=ORIENTED_EDGE('',*,*,#5677,.F.);
#7321=ORIENTED_EDGE('',*,*,#5702,.T.);
#7322=ORIENTED_EDGE('',*,*,#5632,.F.);
#7323=ORIENTED_EDGE('',*,*,#5674,.F.);
#7324=ORIENTED_EDGE('',*,*,#5634,.F.);
#7325=ORIENTED_EDGE('',*,*,#5703,.T.);
#7326=ORIENTED_EDGE('',*,*,#5675,.T.);
#7327=ORIENTED_EDGE('',*,*,#5659,.F.);
#7328=ORIENTED_EDGE('',*,*,#5633,.F.);
#7329=ORIENTED_EDGE('',*,*,#5702,.F.);
#7330=ORIENTED_EDGE('',*,*,#5676,.F.);
#7331=ORIENTED_EDGE('',*,*,#5703,.F.);
#7332=ORIENTED_EDGE('',*,*,#5615,.T.);
#7333=ORIENTED_EDGE('',*,*,#5704,.T.);
#7334=ORIENTED_EDGE('',*,*,#5663,.T.);
#7335=ORIENTED_EDGE('',*,*,#5705,.T.);
#7336=ORIENTED_EDGE('',*,*,#5602,.F.);
#7337=ORIENTED_EDGE('',*,*,#5596,.F.);
#7338=ORIENTED_EDGE('',*,*,#5624,.T.);
#7339=ORIENTED_EDGE('',*,*,#5664,.F.);
#7340=ORIENTED_EDGE('',*,*,#5704,.F.);
#7341=ORIENTED_EDGE('',*,*,#5614,.T.);
#7342=ORIENTED_EDGE('',*,*,#5628,.T.);
#7343=ORIENTED_EDGE('',*,*,#5616,.F.);
#7344=ORIENTED_EDGE('',*,*,#5705,.F.);
#7345=ORIENTED_EDGE('',*,*,#5662,.T.);
#10150=CYLINDRICAL_SURFACE('',#11161,2.);
#10151=CYLINDRICAL_SURFACE('',#11164,2.);
#10152=CYLINDRICAL_SURFACE('',#11167,4.);
#10153=CYLINDRICAL_SURFACE('',#11170,2.25);
#10154=CYLINDRICAL_SURFACE('',#11173,4.);
#10155=CYLINDRICAL_SURFACE('',#11176,2.25);
#10156=CYLINDRICAL_SURFACE('',#11179,7.00000000000001);
#10157=CYLINDRICAL_SURFACE('',#11182,10.);
#10158=CYLINDRICAL_SURFACE('',#11185,11.1);
#10159=CYLINDRICAL_SURFACE('',#11196,12.5);
#10160=CYLINDRICAL_SURFACE('',#11209,2.);
#10161=CYLINDRICAL_SURFACE('',#11210,2.);
#10362=ADVANCED_FACE('',(#725),#10150,.F.);
#10363=ADVANCED_FACE('',(#726),#10151,.F.);
#10364=ADVANCED_FACE('',(#727),#10152,.F.);
#10365=ADVANCED_FACE('',(#728),#10153,.F.);
#10366=ADVANCED_FACE('',(#729),#10154,.F.);
#10367=ADVANCED_FACE('',(#730),#10155,.F.);
#10368=ADVANCED_FACE('',(#731),#10156,.F.);
#10369=ADVANCED_FACE('',(#732),#10157,.F.);
#10370=ADVANCED_FACE('',(#733),#10158,.F.);
#10371=ADVANCED_FACE('',(#734),#381,.F.);
#10372=ADVANCED_FACE('',(#735),#382,.F.);
#10373=ADVANCED_FACE('',(#736),#383,.F.);
#10374=ADVANCED_FACE('',(#737,#251,#252,#253),#384,.F.);
#10375=ADVANCED_FACE('',(#738),#385,.T.);
#10376=ADVANCED_FACE('',(#739),#10159,.T.);
#10377=ADVANCED_FACE('',(#740),#386,.T.);
#10378=ADVANCED_FACE('',(#741),#387,.F.);
#10379=ADVANCED_FACE('',(#742),#388,.F.);
#10380=ADVANCED_FACE('',(#743,#254,#255,#256,#257,#258),#389,.T.);
#10381=ADVANCED_FACE('',(#744,#259),#390,.T.);
#10382=ADVANCED_FACE('',(#745,#260),#391,.T.);
#10383=ADVANCED_FACE('',(#746),#392,.F.);
#10384=ADVANCED_FACE('',(#747),#393,.F.);
#10385=ADVANCED_FACE('',(#748),#394,.T.);
#10386=ADVANCED_FACE('',(#749),#10160,.T.);
#10387=ADVANCED_FACE('',(#750),#10161,.T.);
#10388=ADVANCED_FACE('',(#751,#261),#395,.F.);
#10389=ADVANCED_FACE('',(#752,#262),#396,.F.);
#10390=ADVANCED_FACE('',(#753),#397,.F.);
#10391=ADVANCED_FACE('',(#754),#398,.F.);
#10392=ADVANCED_FACE('',(#755),#399,.F.);
#10393=ADVANCED_FACE('',(#756),#400,.F.);
#10394=ADVANCED_FACE('',(#757),#401,.F.);
#10395=ADVANCED_FACE('',(#758),#402,.F.);
#10396=ADVANCED_FACE('',(#759,#263),#403,.F.);
#10397=ADVANCED_FACE('',(#760),#404,.F.);
#10398=ADVANCED_FACE('',(#761),#405,.F.);
#10399=ADVANCED_FACE('',(#762),#406,.F.);
#10400=ADVANCED_FACE('',(#763),#407,.F.);
#10401=ADVANCED_FACE('',(#764),#408,.F.);
#10402=ADVANCED_FACE('',(#765),#409,.F.);
#10403=ADVANCED_FACE('',(#766,#264),#410,.T.);
#10404=ADVANCED_FACE('',(#767),#411,.T.);
#10405=ADVANCED_FACE('',(#768),#412,.T.);
#10406=ADVANCED_FACE('',(#769),#413,.F.);
#10407=ADVANCED_FACE('',(#770,#265,#266),#414,.T.);
#10408=ADVANCED_FACE('',(#771),#415,.F.);
#10409=ADVANCED_FACE('',(#772),#416,.F.);
#10958=CLOSED_SHELL('',(#10362,#10363,#10364,#10365,#10366,#10367,#10368,
#10369,#10370,#10371,#10372,#10373,#10374,#10375,#10376,#10377,#10378,#10379,
#10380,#10381,#10382,#10383,#10384,#10385,#10386,#10387,#10388,#10389,#10390,
#10391,#10392,#10393,#10394,#10395,#10396,#10397,#10398,#10399,#10400,#10401,
#10402,#10403,#10404,#10405,#10406,#10407,#10408,#10409));
#11160=AXIS2_PLACEMENT_3D('',#15606,#12305,#12306);
#11161=AXIS2_PLACEMENT_3D('',#15607,#12307,#12308);
#11162=AXIS2_PLACEMENT_3D('',#15609,#12309,#12310);
#11163=AXIS2_PLACEMENT_3D('',#15612,#12312,#12313);
#11164=AXIS2_PLACEMENT_3D('',#15613,#12314,#12315);
#11165=AXIS2_PLACEMENT_3D('',#15615,#12316,#12317);
#11166=AXIS2_PLACEMENT_3D('',#15618,#12319,#12320);
#11167=AXIS2_PLACEMENT_3D('',#15619,#12321,#12322);
#11168=AXIS2_PLACEMENT_3D('',#15621,#12323,#12324);
#11169=AXIS2_PLACEMENT_3D('',#15624,#12326,#12327);
#11170=AXIS2_PLACEMENT_3D('',#15625,#12328,#12329);
#11171=AXIS2_PLACEMENT_3D('',#15627,#12330,#12331);
#11172=AXIS2_PLACEMENT_3D('',#15630,#12333,#12334);
#11173=AXIS2_PLACEMENT_3D('',#15631,#12335,#12336);
#11174=AXIS2_PLACEMENT_3D('',#15633,#12337,#12338);
#11175=AXIS2_PLACEMENT_3D('',#15636,#12340,#12341);
#11176=AXIS2_PLACEMENT_3D('',#15637,#12342,#12343);
#11177=AXIS2_PLACEMENT_3D('',#15639,#12344,#12345);
#11178=AXIS2_PLACEMENT_3D('',#15642,#12347,#12348);
#11179=AXIS2_PLACEMENT_3D('',#15643,#12349,#12350);
#11180=AXIS2_PLACEMENT_3D('',#15645,#12351,#12352);
#11181=AXIS2_PLACEMENT_3D('',#15648,#12354,#12355);
#11182=AXIS2_PLACEMENT_3D('',#15649,#12356,#12357);
#11183=AXIS2_PLACEMENT_3D('',#15651,#12358,#12359);
#11184=AXIS2_PLACEMENT_3D('',#15654,#12361,#12362);
#11185=AXIS2_PLACEMENT_3D('',#15655,#12363,#12364);
#11186=AXIS2_PLACEMENT_3D('',#15657,#12365,#12366);
#11187=AXIS2_PLACEMENT_3D('',#15660,#12368,#12369);
#11188=AXIS2_PLACEMENT_3D('',#15661,#12370,#12371);
#11189=AXIS2_PLACEMENT_3D('',#15682,#12382,#12383);
#11190=AXIS2_PLACEMENT_3D('',#15688,#12386,#12387);
#11191=AXIS2_PLACEMENT_3D('',#15690,#12389,#12390);
#11192=AXIS2_PLACEMENT_3D('',#15696,#12393,#12394);
#11193=AXIS2_PLACEMENT_3D('',#15698,#12396,#12397);
#11194=AXIS2_PLACEMENT_3D('',#15709,#12402,#12403);
#11195=AXIS2_PLACEMENT_3D('',#15738,#12419,#12420);
#11196=AXIS2_PLACEMENT_3D('',#15744,#12424,#12425);
#11197=AXIS2_PLACEMENT_3D('',#15747,#12427,#12428);
#11198=AXIS2_PLACEMENT_3D('',#15748,#12429,#12430);
#11199=AXIS2_PLACEMENT_3D('',#15755,#12435,#12436);
#11200=AXIS2_PLACEMENT_3D('',#15766,#12443,#12444);
#11201=AXIS2_PLACEMENT_3D('',#15770,#12447,#12448);
#11202=AXIS2_PLACEMENT_3D('',#15771,#12449,#12450);
#11203=AXIS2_PLACEMENT_3D('',#15772,#12451,#12452);
#11204=AXIS2_PLACEMENT_3D('',#15773,#12453,#12454);
#11205=AXIS2_PLACEMENT_3D('',#15774,#12455,#12456);
#11206=AXIS2_PLACEMENT_3D('',#15775,#12457,#12458);
#11207=AXIS2_PLACEMENT_3D('',#15779,#12461,#12462);
#11208=AXIS2_PLACEMENT_3D('',#15783,#12465,#12466);
#11209=AXIS2_PLACEMENT_3D('',#15789,#12470,#12471);
#11210=AXIS2_PLACEMENT_3D('',#15790,#12472,#12473);
#11211=AXIS2_PLACEMENT_3D('',#15791,#12474,#12475);
#11212=AXIS2_PLACEMENT_3D('',#15792,#12476,#12477);
#11213=AXIS2_PLACEMENT_3D('',#15793,#12478,#12479);
#11214=AXIS2_PLACEMENT_3D('',#15799,#12483,#12484);
#11215=AXIS2_PLACEMENT_3D('',#15803,#12487,#12488);
#11216=AXIS2_PLACEMENT_3D('',#15807,#12491,#12492);
#11217=AXIS2_PLACEMENT_3D('',#15811,#12495,#12496);
#11218=AXIS2_PLACEMENT_3D('',#15815,#12499,#12500);
#11219=AXIS2_PLACEMENT_3D('',#15817,#12502,#12503);
#11220=AXIS2_PLACEMENT_3D('',#15818,#12504,#12505);
#11221=AXIS2_PLACEMENT_3D('',#15824,#12509,#12510);
#11222=AXIS2_PLACEMENT_3D('',#15828,#12513,#12514);
#11223=AXIS2_PLACEMENT_3D('',#15832,#12517,#12518);
#11224=AXIS2_PLACEMENT_3D('',#15836,#12521,#12522);
#11225=AXIS2_PLACEMENT_3D('',#15840,#12525,#12526);
#11226=AXIS2_PLACEMENT_3D('',#15842,#12528,#12529);
#11227=AXIS2_PLACEMENT_3D('',#15843,#12530,#12531);
#11228=AXIS2_PLACEMENT_3D('',#15845,#12533,#12534);
#11229=AXIS2_PLACEMENT_3D('',#15847,#12536,#12537);
#11230=AXIS2_PLACEMENT_3D('',#15848,#12538,#12539);
#11231=AXIS2_PLACEMENT_3D('',#15851,#12542,#12543);
#11232=AXIS2_PLACEMENT_3D('',#15852,#12544,#12545);
#12305=DIRECTION('axis',(0.,0.,1.));
#12306=DIRECTION('refdir',(1.,0.,0.));
#12307=DIRECTION('center_axis',(0.,0.,-1.));
#12308=DIRECTION('ref_axis',(-1.,0.,0.));
#12309=DIRECTION('center_axis',(0.,0.,-1.));
#12310=DIRECTION('ref_axis',(-1.,0.,0.));
#12311=DIRECTION('',(0.,0.,-1.));
#12312=DIRECTION('center_axis',(0.,0.,-1.));
#12313=DIRECTION('ref_axis',(-1.,0.,0.));
#12314=DIRECTION('center_axis',(0.,0.,-1.));
#12315=DIRECTION('ref_axis',(-1.,0.,0.));
#12316=DIRECTION('center_axis',(0.,0.,-1.));
#12317=DIRECTION('ref_axis',(-1.,0.,0.));
#12318=DIRECTION('',(0.,0.,-1.));
#12319=DIRECTION('center_axis',(0.,0.,-1.));
#12320=DIRECTION('ref_axis',(-1.,0.,0.));
#12321=DIRECTION('center_axis',(0.,0.,1.));
#12322=DIRECTION('ref_axis',(1.,0.,0.));
#12323=DIRECTION('center_axis',(0.,0.,1.));
#12324=DIRECTION('ref_axis',(1.,0.,0.));
#12325=DIRECTION('',(0.,0.,1.));
#12326=DIRECTION('center_axis',(0.,0.,1.));
#12327=DIRECTION('ref_axis',(1.,0.,0.));
#12328=DIRECTION('center_axis',(0.,0.,1.));
#12329=DIRECTION('ref_axis',(1.,0.,0.));
#12330=DIRECTION('center_axis',(0.,-1.15648231731787E-16,-1.));
#12331=DIRECTION('ref_axis',(0.,1.,-1.15648231731787E-16));
#12332=DIRECTION('',(0.,0.,1.));
#12333=DIRECTION('center_axis',(0.,0.,1.));
#12334=DIRECTION('ref_axis',(1.,0.,0.));
#12335=DIRECTION('center_axis',(0.,0.,1.));
#12336=DIRECTION('ref_axis',(1.,0.,0.));
#12337=DIRECTION('center_axis',(0.,0.,1.));
#12338=DIRECTION('ref_axis',(1.,0.,0.));
#12339=DIRECTION('',(0.,0.,1.));
#12340=DIRECTION('center_axis',(0.,0.,1.));
#12341=DIRECTION('ref_axis',(1.,0.,0.));
#12342=DIRECTION('center_axis',(0.,0.,1.));
#12343=DIRECTION('ref_axis',(1.,0.,0.));
#12344=DIRECTION('center_axis',(0.,-1.15648231731787E-16,-1.));
#12345=DIRECTION('ref_axis',(0.,1.,-1.15648231731787E-16));
#12346=DIRECTION('',(0.,0.,1.));
#12347=DIRECTION('center_axis',(0.,0.,1.));
#12348=DIRECTION('ref_axis',(1.,0.,0.));
#12349=DIRECTION('center_axis',(0.,0.,-1.));
#12350=DIRECTION('ref_axis',(-1.,0.,0.));
#12351=DIRECTION('center_axis',(0.,0.,-1.));
#12352=DIRECTION('ref_axis',(-1.,0.,0.));
#12353=DIRECTION('',(0.,0.,-1.));
#12354=DIRECTION('center_axis',(0.,0.,-1.));
#12355=DIRECTION('ref_axis',(-1.,0.,0.));
#12356=DIRECTION('center_axis',(0.,0.,-1.));
#12357=DIRECTION('ref_axis',(-1.,0.,0.));
#12358=DIRECTION('center_axis',(0.,0.,-1.));
#12359=DIRECTION('ref_axis',(-1.,0.,0.));
#12360=DIRECTION('',(0.,0.,-1.));
#12361=DIRECTION('center_axis',(0.,0.,-1.));
#12362=DIRECTION('ref_axis',(-1.,0.,0.));
#12363=DIRECTION('center_axis',(0.,0.,-1.));
#12364=DIRECTION('ref_axis',(-1.,0.,0.));
#12365=DIRECTION('center_axis',(0.,0.,-1.));
#12366=DIRECTION('ref_axis',(-1.,0.,0.));
#12367=DIRECTION('',(0.,0.,-1.));
#12368=DIRECTION('center_axis',(0.,0.,-1.));
#12369=DIRECTION('ref_axis',(-1.,0.,0.));
#12370=DIRECTION('center_axis',(1.,0.,0.));
#12371=DIRECTION('ref_axis',(0.,0.,-1.));
#12372=DIRECTION('',(0.,1.15648231731787E-16,1.));
#12373=DIRECTION('',(0.,-1.,1.09792625061823E-16));
#12374=DIRECTION('',(0.,1.15648231731787E-16,1.));
#12375=DIRECTION('',(0.,1.,-1.15648231731787E-16));
#12376=DIRECTION('',(0.,0.,-1.));
#12377=DIRECTION('',(0.,1.,0.));
#12378=DIRECTION('',(0.,0.,1.));
#12379=DIRECTION('',(0.,1.,0.));
#12380=DIRECTION('',(0.,0.,1.));
#12381=DIRECTION('',(0.,1.,-1.15648231731787E-16));
#12382=DIRECTION('center_axis',(0.,1.15648231731787E-16,1.));
#12383=DIRECTION('ref_axis',(0.,-1.,1.15648231731787E-16));
#12384=DIRECTION('',(-1.,0.,0.));
#12385=DIRECTION('',(-1.,0.,0.));
#12386=DIRECTION('center_axis',(0.,-1.15648231731787E-16,-1.));
#12387=DIRECTION('ref_axis',(0.,-1.,1.15648231731787E-16));
#12388=DIRECTION('',(0.,1.,-1.15648231731787E-16));
#12389=DIRECTION('center_axis',(0.,1.15648231731787E-16,1.));
#12390=DIRECTION('ref_axis',(0.,-1.,1.15648231731787E-16));
#12391=DIRECTION('',(1.,0.,0.));
#12392=DIRECTION('',(0.,1.,-1.15648231731787E-16));
#12393=DIRECTION('center_axis',(0.,-1.15648231731787E-16,-1.));
#12394=DIRECTION('ref_axis',(0.,-1.,1.15648231731787E-16));
#12395=DIRECTION('',(-1.,0.,0.));
#12396=DIRECTION('center_axis',(0.,0.,1.));
#12397=DIRECTION('ref_axis',(1.,0.,0.));
#12398=DIRECTION('',(1.,0.,0.));
#12399=DIRECTION('',(0.86602540378444,0.499999999999998,0.));
#12400=DIRECTION('',(0.,1.,0.));
#12401=DIRECTION('',(1.,0.,0.));
#12402=DIRECTION('center_axis',(0.,0.,1.));
#12403=DIRECTION('ref_axis',(1.,0.,0.));
#12404=DIRECTION('',(-0.977786581118157,-0.209602962253079,0.));
#12405=DIRECTION('',(-0.977786581118157,-0.209602962253078,0.));
#12406=DIRECTION('',(0.,-1.,0.));
#12407=DIRECTION('',(0.,-1.,0.));
#12408=DIRECTION('',(0.866025403784439,-0.499999999999999,0.));
#12409=DIRECTION('',(0.866025403784438,0.500000000000001,0.));
#12410=DIRECTION('',(0.,1.,0.));
#12411=DIRECTION('',(-0.866025403784438,0.500000000000001,0.));
#12412=DIRECTION('',(-0.866025403784439,-0.499999999999999,0.));
#12413=DIRECTION('',(0.,1.,0.));
#12414=DIRECTION('',(-0.866025403784438,0.500000000000001,0.));
#12415=DIRECTION('',(-0.866025403784439,-0.499999999999999,0.));
#12416=DIRECTION('',(0.,-1.,0.));
#12417=DIRECTION('',(0.866025403784439,-0.499999999999999,0.));
#12418=DIRECTION('',(0.866025403784438,0.500000000000001,0.));
#12419=DIRECTION('center_axis',(0.209602962253079,-0.977786581118157,0.));
#12420=DIRECTION('ref_axis',(0.977786581118157,0.209602962253079,0.));
#12421=DIRECTION('',(0.,0.,-1.));
#12422=DIRECTION('',(-0.977786581118157,-0.209602962253079,0.));
#12423=DIRECTION('',(0.,0.,-1.));
#12424=DIRECTION('center_axis',(0.,0.,-1.));
#12425=DIRECTION('ref_axis',(0.99443113917409,0.105388374315774,0.));
#12426=DIRECTION('',(0.,0.,-1.));
#12427=DIRECTION('center_axis',(0.,0.,1.));
#12428=DIRECTION('ref_axis',(1.,0.,0.));
#12429=DIRECTION('center_axis',(0.,1.,0.));
#12430=DIRECTION('ref_axis',(0.,0.,1.));
#12431=DIRECTION('',(0.,0.,1.));
#12432=DIRECTION('',(1.,0.,0.));
#12433=DIRECTION('',(0.,0.,-1.));
#12434=DIRECTION('',(-1.,0.,0.));
#12435=DIRECTION('center_axis',(1.,0.,0.));
#12436=DIRECTION('ref_axis',(0.,0.,-1.));
#12437=DIRECTION('',(0.,0.,-1.));
#12438=DIRECTION('',(0.,1.15648231731787E-16,1.));
#12439=DIRECTION('',(0.,1.,-1.09792625061823E-16));
#12440=DIRECTION('',(0.,1.15648231731787E-16,1.));
#12441=DIRECTION('',(0.,0.,1.));
#12442=DIRECTION('',(0.,-1.,0.));
#12443=DIRECTION('center_axis',(-9.91270557701033E-17,1.,0.));
#12444=DIRECTION('ref_axis',(-1.,-9.91270557701033E-17,0.));
#12445=DIRECTION('',(0.,0.,-1.));
#12446=DIRECTION('',(1.,9.91270557701033E-17,0.));
#12447=DIRECTION('center_axis',(0.,0.,1.));
#12448=DIRECTION('ref_axis',(1.,0.,0.));
#12449=DIRECTION('center_axis',(0.,0.,1.));
#12450=DIRECTION('ref_axis',(1.,0.,0.));
#12451=DIRECTION('center_axis',(0.,0.,1.));
#12452=DIRECTION('ref_axis',(1.,0.,0.));
#12453=DIRECTION('center_axis',(0.,0.,-1.));
#12454=DIRECTION('ref_axis',(-1.,0.,0.));
#12455=DIRECTION('center_axis',(0.,0.,-1.));
#12456=DIRECTION('ref_axis',(-1.,0.,0.));
#12457=DIRECTION('center_axis',(-0.209602962253078,0.977786581118157,0.));
#12458=DIRECTION('ref_axis',(-0.977786581118157,-0.209602962253078,0.));
#12459=DIRECTION('',(-0.977786581118157,-0.209602962253078,0.));
#12460=DIRECTION('',(0.,0.,1.));
#12461=DIRECTION('center_axis',(-1.,0.,0.));
#12462=DIRECTION('ref_axis',(0.,0.,1.));
#12463=DIRECTION('',(0.,-1.,0.));
#12464=DIRECTION('',(0.,0.,1.));
#12465=DIRECTION('center_axis',(0.,0.,-1.));
#12466=DIRECTION('ref_axis',(-1.,0.,0.));
#12467=DIRECTION('',(0.,1.,0.));
#12468=DIRECTION('',(-0.86602540378444,-0.499999999999998,0.));
#12469=DIRECTION('',(-1.,0.,0.));
#12470=DIRECTION('center_axis',(0.,0.,-1.));
#12471=DIRECTION('ref_axis',(-1.,0.,0.));
#12472=DIRECTION('center_axis',(0.,0.,1.));
#12473=DIRECTION('ref_axis',(1.,0.,0.));
#12474=DIRECTION('center_axis',(0.,0.,-1.));
#12475=DIRECTION('ref_axis',(-1.,0.,0.));
#12476=DIRECTION('center_axis',(0.,0.,-1.));
#12477=DIRECTION('ref_axis',(-1.,0.,0.));
#12478=DIRECTION('center_axis',(-0.500000000000001,-0.866025403784438,0.));
#12479=DIRECTION('ref_axis',(0.866025403784438,-0.500000000000001,0.));
#12480=DIRECTION('',(0.,0.,-1.));
#12481=DIRECTION('',(-0.866025403784438,0.500000000000001,0.));
#12482=DIRECTION('',(0.,0.,-1.));
#12483=DIRECTION('center_axis',(0.499999999999999,-0.866025403784439,0.));
#12484=DIRECTION('ref_axis',(0.866025403784439,0.499999999999999,0.));
#12485=DIRECTION('',(-0.866025403784439,-0.499999999999999,0.));
#12486=DIRECTION('',(0.,0.,-1.));
#12487=DIRECTION('center_axis',(1.,0.,0.));
#12488=DIRECTION('ref_axis',(0.,0.,-1.));
#12489=DIRECTION('',(0.,-1.,0.));
#12490=DIRECTION('',(0.,0.,-1.));
#12491=DIRECTION('center_axis',(0.499999999999999,0.866025403784439,0.));
#12492=DIRECTION('ref_axis',(-0.866025403784439,0.499999999999999,0.));
#12493=DIRECTION('',(0.866025403784439,-0.499999999999999,0.));
#12494=DIRECTION('',(0.,0.,-1.));
#12495=DIRECTION('center_axis',(-0.500000000000001,0.866025403784438,0.));
#12496=DIRECTION('ref_axis',(-0.866025403784438,-0.500000000000001,0.));
#12497=DIRECTION('',(0.866025403784438,0.500000000000001,0.));
#12498=DIRECTION('',(0.,0.,-1.));
#12499=DIRECTION('center_axis',(-1.,0.,0.));
#12500=DIRECTION('ref_axis',(0.,0.,1.));
#12501=DIRECTION('',(0.,1.,0.));
#12502=DIRECTION('center_axis',(0.,0.,1.));
#12503=DIRECTION('ref_axis',(1.,0.,0.));
#12504=DIRECTION('center_axis',(0.499999999999999,0.866025403784439,0.));
#12505=DIRECTION('ref_axis',(-0.866025403784439,0.499999999999999,0.));
#12506=DIRECTION('',(0.,0.,-1.));
#12507=DIRECTION('',(0.866025403784439,-0.499999999999999,0.));
#12508=DIRECTION('',(0.,0.,-1.));
#12509=DIRECTION('center_axis',(-0.500000000000001,0.866025403784438,0.));
#12510=DIRECTION('ref_axis',(-0.866025403784438,-0.500000000000001,0.));
#12511=DIRECTION('',(0.866025403784438,0.500000000000001,0.));
#12512=DIRECTION('',(0.,0.,-1.));
#12513=DIRECTION('center_axis',(-1.,0.,0.));
#12514=DIRECTION('ref_axis',(0.,0.,1.));
#12515=DIRECTION('',(0.,1.,0.));
#12516=DIRECTION('',(0.,0.,-1.));
#12517=DIRECTION('center_axis',(-0.500000000000001,-0.866025403784438,0.));
#12518=DIRECTION('ref_axis',(0.866025403784438,-0.500000000000001,0.));
#12519=DIRECTION('',(-0.866025403784438,0.500000000000001,0.));
#12520=DIRECTION('',(0.,0.,-1.));
#12521=DIRECTION('center_axis',(0.499999999999999,-0.866025403784439,0.));
#12522=DIRECTION('ref_axis',(0.866025403784439,0.499999999999999,0.));
#12523=DIRECTION('',(-0.866025403784439,-0.499999999999999,0.));
#12524=DIRECTION('',(0.,0.,-1.));
#12525=DIRECTION('center_axis',(1.,0.,0.));
#12526=DIRECTION('ref_axis',(0.,0.,-1.));
#12527=DIRECTION('',(0.,-1.,0.));
#12528=DIRECTION('center_axis',(0.,0.,-1.));
#12529=DIRECTION('ref_axis',(-1.,0.,0.));
#12530=DIRECTION('center_axis',(0.,-1.,0.));
#12531=DIRECTION('ref_axis',(0.,0.,-1.));
#12532=DIRECTION('',(0.,0.,1.));
#12533=DIRECTION('center_axis',(1.,0.,0.));
#12534=DIRECTION('ref_axis',(0.,0.,-1.));
#12535=DIRECTION('',(0.,0.,-1.));
#12536=DIRECTION('center_axis',(-0.499999999999998,0.86602540378444,0.));
#12537=DIRECTION('ref_axis',(0.,0.,-1.));
#12538=DIRECTION('center_axis',(0.,-1.09792625061823E-16,-1.));
#12539=DIRECTION('ref_axis',(0.,1.,-1.09792625061823E-16));
#12540=DIRECTION('',(-1.,0.,0.));
#12541=DIRECTION('',(1.,0.,0.));
#12542=DIRECTION('center_axis',(0.,1.,-1.15648231731787E-16));
#12543=DIRECTION('ref_axis',(0.,1.15648231731787E-16,1.));
#12544=DIRECTION('center_axis',(0.,-1.,1.15648231731787E-16));
#12545=DIRECTION('ref_axis',(0.,-1.15648231731787E-16,-1.));
#15606=CARTESIAN_POINT('',(0.,0.,0.));
#15607=CARTESIAN_POINT('Origin',(198.2,9.50000000000001,9.));
#15608=CARTESIAN_POINT('',(200.2,9.50000000000001,9.));
#15609=CARTESIAN_POINT('Origin',(198.2,9.50000000000001,9.));
#15610=CARTESIAN_POINT('',(200.2,9.50000000000001,3.));
#15611=CARTESIAN_POINT('',(200.2,9.50000000000001,9.));
#15612=CARTESIAN_POINT('Origin',(198.2,9.50000000000001,3.));
#15613=CARTESIAN_POINT('Origin',(198.2,-4.49999999999994,9.));
#15614=CARTESIAN_POINT('',(200.2,-4.49999999999994,9.));
#15615=CARTESIAN_POINT('Origin',(198.2,-4.49999999999994,9.));
#15616=CARTESIAN_POINT('',(200.2,-4.49999999999994,3.));
#15617=CARTESIAN_POINT('',(200.2,-4.49999999999994,9.));
#15618=CARTESIAN_POINT('Origin',(198.2,-4.49999999999994,3.));
#15619=CARTESIAN_POINT('Origin',(162.5,0.,9.));
#15620=CARTESIAN_POINT('',(158.5,-4.89858719658942E-16,4.6));
#15621=CARTESIAN_POINT('Origin',(162.5,0.,4.6));
#15622=CARTESIAN_POINT('',(158.5,-4.89858719658942E-16,9.));
#15623=CARTESIAN_POINT('',(158.5,-4.89858719658942E-16,9.));
#15624=CARTESIAN_POINT('Origin',(162.5,0.,9.));
#15625=CARTESIAN_POINT('Origin',(162.5,0.,9.));
#15626=CARTESIAN_POINT('',(160.25,-2.75545529808155E-16,1.));
#15627=CARTESIAN_POINT('Origin',(162.5,-2.31296463463574E-16,1.));
#15628=CARTESIAN_POINT('',(160.25,-2.75545529808155E-16,4.6));
#15629=CARTESIAN_POINT('',(160.25,-2.75545529808155E-16,9.));
#15630=CARTESIAN_POINT('Origin',(162.5,0.,4.6));
#15631=CARTESIAN_POINT('Origin',(182.5,0.,9.));
#15632=CARTESIAN_POINT('',(178.5,-4.89858719658942E-16,4.6));
#15633=CARTESIAN_POINT('Origin',(182.5,0.,4.6));
#15634=CARTESIAN_POINT('',(178.5,-4.89858719658942E-16,9.));
#15635=CARTESIAN_POINT('',(178.5,-4.89858719658942E-16,9.));
#15636=CARTESIAN_POINT('Origin',(182.5,0.,9.));
#15637=CARTESIAN_POINT('Origin',(182.5,0.,9.));
#15638=CARTESIAN_POINT('',(180.25,-2.75545529808155E-16,1.));
#15639=CARTESIAN_POINT('Origin',(182.5,-2.31296463463574E-16,1.));
#15640=CARTESIAN_POINT('',(180.25,-2.75545529808155E-16,4.6));
#15641=CARTESIAN_POINT('',(180.25,-2.75545529808155E-16,9.));
#15642=CARTESIAN_POINT('Origin',(182.5,0.,4.6));
#15643=CARTESIAN_POINT('Origin',(212.,2.50000000000003,9.));
#15644=CARTESIAN_POINT('',(219.,2.50000000000003,9.));
#15645=CARTESIAN_POINT('Origin',(212.,2.50000000000003,9.));
#15646=CARTESIAN_POINT('',(219.,2.50000000000003,8.));
#15647=CARTESIAN_POINT('',(219.,2.50000000000003,9.));
#15648=CARTESIAN_POINT('Origin',(212.,2.50000000000003,8.));
#15649=CARTESIAN_POINT('Origin',(212.,2.50000000000003,8.));
#15650=CARTESIAN_POINT('',(222.,2.50000000000003,8.));
#15651=CARTESIAN_POINT('Origin',(212.,2.50000000000003,8.));
#15652=CARTESIAN_POINT('',(222.,2.50000000000003,7.));
#15653=CARTESIAN_POINT('',(222.,2.50000000000003,8.));
#15654=CARTESIAN_POINT('Origin',(212.,2.50000000000003,7.));
#15655=CARTESIAN_POINT('Origin',(212.,2.50000000000003,7.));
#15656=CARTESIAN_POINT('',(223.1,2.50000000000003,7.));
#15657=CARTESIAN_POINT('Origin',(212.,2.50000000000003,7.));
#15658=CARTESIAN_POINT('',(223.1,2.50000000000003,0.));
#15659=CARTESIAN_POINT('',(223.1,2.50000000000003,7.));
#15660=CARTESIAN_POINT('Origin',(212.,2.50000000000003,0.));
#15661=CARTESIAN_POINT('Origin',(190.,0.,-10.));
#15662=CARTESIAN_POINT('',(190.,-3.95,1.));
#15663=CARTESIAN_POINT('',(190.,-3.95,3.));
#15664=CARTESIAN_POINT('',(190.,-3.95,1.));
#15665=CARTESIAN_POINT('',(190.,3.95,1.));
#15666=CARTESIAN_POINT('',(190.,-3.95,1.));
#15667=CARTESIAN_POINT('',(190.,3.95,3.));
#15668=CARTESIAN_POINT('',(190.,3.95,1.));
#15669=CARTESIAN_POINT('',(190.,15.,3.));
#15670=CARTESIAN_POINT('',(190.,15.,3.));
#15671=CARTESIAN_POINT('',(190.,15.,-10.));
#15672=CARTESIAN_POINT('',(190.,15.,3.));
#15673=CARTESIAN_POINT('',(190.,-13.9772819352292,-10.));
#15674=CARTESIAN_POINT('',(190.,0.,-10.));
#15675=CARTESIAN_POINT('',(190.,-13.9772819352292,0.));
#15676=CARTESIAN_POINT('',(190.,-13.9772819352292,-10.));
#15677=CARTESIAN_POINT('',(190.,-15.,0.));
#15678=CARTESIAN_POINT('',(190.,0.,0.));
#15679=CARTESIAN_POINT('',(190.,-15.,3.));
#15680=CARTESIAN_POINT('',(190.,-15.,3.));
#15681=CARTESIAN_POINT('',(190.,15.,3.));
#15682=CARTESIAN_POINT('Origin',(190.,15.,3.));
#15683=CARTESIAN_POINT('',(155.,-3.94999999999999,3.));
#15684=CARTESIAN_POINT('',(155.,-3.95,3.));
#15685=CARTESIAN_POINT('',(157.,-15.,3.));
#15686=CARTESIAN_POINT('',(190.,-15.,3.));
#15687=CARTESIAN_POINT('',(155.,-13.,3.));
#15688=CARTESIAN_POINT('Origin',(157.,-13.,3.));
#15689=CARTESIAN_POINT('',(155.,15.,3.));
#15690=CARTESIAN_POINT('Origin',(190.,15.,3.));
#15691=CARTESIAN_POINT('',(155.,3.95,3.));
#15692=CARTESIAN_POINT('',(155.,3.95,3.));
#15693=CARTESIAN_POINT('',(155.,13.,3.));
#15694=CARTESIAN_POINT('',(155.,15.,3.));
#15695=CARTESIAN_POINT('',(157.,15.,3.));
#15696=CARTESIAN_POINT('Origin',(157.,13.,3.));
#15697=CARTESIAN_POINT('',(190.,15.,3.));
#15698=CARTESIAN_POINT('Origin',(0.,0.,0.));
#15699=CARTESIAN_POINT('',(195.,13.,0.));
#15700=CARTESIAN_POINT('',(203.5,13.,0.));
#15701=CARTESIAN_POINT('',(190.,13.,0.));
#15702=CARTESIAN_POINT('',(205.,13.8660254037845,0.));
#15703=CARTESIAN_POINT('',(45.2458348754007,-78.3680848350663,0.));
#15704=CARTESIAN_POINT('',(205.,15.,0.));
#15705=CARTESIAN_POINT('',(205.,13.,0.));
#15706=CARTESIAN_POINT('',(212.,15.,0.));
#15707=CARTESIAN_POINT('',(0.,15.,0.));
#15708=CARTESIAN_POINT('',(214.620037028164,-9.72233226397694,0.));
#15709=CARTESIAN_POINT('Origin',(212.,2.50000000000003,0.));
#15710=CARTESIAN_POINT('',(11.4215507970056,-53.2809221054195,0.));
#15711=CARTESIAN_POINT('',(195.,-12.9054582556007,0.));
#15712=CARTESIAN_POINT('',(11.2119478347524,-52.3031355243012,0.));
#15713=CARTESIAN_POINT('',(195.,0.,0.));
#15714=CARTESIAN_POINT('',(201.2,11.2320508075689,0.));
#15715=CARTESIAN_POINT('',(201.2,7.76794919243114,0.));
#15716=CARTESIAN_POINT('',(201.2,11.2320508075689,0.));
#15717=CARTESIAN_POINT('',(198.2,12.9641016151378,0.));
#15718=CARTESIAN_POINT('',(198.2,12.9641016151378,0.));
#15719=CARTESIAN_POINT('',(195.2,11.2320508075689,0.));
#15720=CARTESIAN_POINT('',(195.2,11.2320508075689,0.));
#15721=CARTESIAN_POINT('',(195.2,7.76794919243112,0.));
#15722=CARTESIAN_POINT('',(195.2,7.76794919243112,0.));
#15723=CARTESIAN_POINT('',(198.2,6.03589838486225,0.));
#15724=CARTESIAN_POINT('',(198.2,6.03589838486225,0.));
#15725=CARTESIAN_POINT('',(201.2,7.76794919243114,0.));
#15726=CARTESIAN_POINT('',(195.2,-6.23205080756882,0.));
#15727=CARTESIAN_POINT('',(195.2,-2.76794919243105,0.));
#15728=CARTESIAN_POINT('',(195.2,-2.76794919243105,0.));
#15729=CARTESIAN_POINT('',(198.2,-7.9641016151377,0.));
#15730=CARTESIAN_POINT('',(195.2,-6.23205080756882,0.));
#15731=CARTESIAN_POINT('',(201.2,-6.23205080756883,0.));
#15732=CARTESIAN_POINT('',(198.2,-7.9641016151377,0.));
#15733=CARTESIAN_POINT('',(201.2,-2.76794919243107,0.));
#15734=CARTESIAN_POINT('',(201.2,-6.23205080756883,0.));
#15735=CARTESIAN_POINT('',(198.2,-1.03589838486218,0.));
#15736=CARTESIAN_POINT('',(201.2,-2.76794919243107,0.));
#15737=CARTESIAN_POINT('',(198.2,-1.03589838486218,0.));
#15738=CARTESIAN_POINT('Origin',(11.4215507970056,-53.2809221054195,9.));
#15739=CARTESIAN_POINT('',(214.620037028164,-9.72233226397694,9.));
#15740=CARTESIAN_POINT('',(214.620037028164,-9.72233226397694,9.));
#15741=CARTESIAN_POINT('',(190.,-15.,9.));
#15742=CARTESIAN_POINT('',(11.4215507970056,-53.2809221054195,9.));
#15743=CARTESIAN_POINT('',(190.,-15.,9.));
#15744=CARTESIAN_POINT('Origin',(212.,2.50000000000003,9.));
#15745=CARTESIAN_POINT('',(212.,15.,9.));
#15746=CARTESIAN_POINT('',(212.,15.,9.));
#15747=CARTESIAN_POINT('Origin',(212.,2.50000000000003,9.));
#15748=CARTESIAN_POINT('Origin',(0.,15.,9.));
#15749=CARTESIAN_POINT('',(157.,15.,9.));
#15750=CARTESIAN_POINT('',(157.,15.,9.));
#15751=CARTESIAN_POINT('',(0.,15.,9.));
#15752=CARTESIAN_POINT('',(205.,15.,-10.));
#15753=CARTESIAN_POINT('',(205.,15.,0.));
#15754=CARTESIAN_POINT('',(190.,15.,-10.));
#15755=CARTESIAN_POINT('Origin',(155.,0.,9.));
#15756=CARTESIAN_POINT('',(155.,13.,9.));
#15757=CARTESIAN_POINT('',(155.,13.,0.));
#15758=CARTESIAN_POINT('',(155.,3.95,1.));
#15759=CARTESIAN_POINT('',(155.,3.95,1.));
#15760=CARTESIAN_POINT('',(155.,-3.95,1.));
#15761=CARTESIAN_POINT('',(155.,-3.95,1.));
#15762=CARTESIAN_POINT('',(155.,-3.95,1.));
#15763=CARTESIAN_POINT('',(155.,-13.,9.));
#15764=CARTESIAN_POINT('',(155.,-13.,9.));
#15765=CARTESIAN_POINT('',(155.,0.,9.));
#15766=CARTESIAN_POINT('Origin',(1.48690583655155E-15,-15.,9.));
#15767=CARTESIAN_POINT('',(157.,-15.,9.));
#15768=CARTESIAN_POINT('',(157.,-15.,9.));
#15769=CARTESIAN_POINT('',(1.48690583655155E-15,-15.,9.));
#15770=CARTESIAN_POINT('Origin',(0.,0.,9.));
#15771=CARTESIAN_POINT('Origin',(157.,-13.,9.));
#15772=CARTESIAN_POINT('Origin',(157.,13.,9.));
#15773=CARTESIAN_POINT('Origin',(212.,2.50000000000003,7.));
#15774=CARTESIAN_POINT('Origin',(212.,2.50000000000003,8.));
#15775=CARTESIAN_POINT('Origin',(11.2119478347524,-52.3031355243012,-10.));
#15776=CARTESIAN_POINT('',(195.,-12.9054582556007,-10.));
#15777=CARTESIAN_POINT('',(11.2119478347524,-52.3031355243012,-10.));
#15778=CARTESIAN_POINT('',(195.,-12.9054582556007,-10.));
#15779=CARTESIAN_POINT('Origin',(195.,0.,-10.));
#15780=CARTESIAN_POINT('',(195.,13.,-10.));
#15781=CARTESIAN_POINT('',(195.,0.,-10.));
#15782=CARTESIAN_POINT('',(195.,13.,-10.));
#15783=CARTESIAN_POINT('Origin',(0.,0.,-10.));
#15784=CARTESIAN_POINT('',(205.,13.8660254037845,-10.));
#15785=CARTESIAN_POINT('',(205.,13.,-10.));
#15786=CARTESIAN_POINT('',(203.5,13.,-10.));
#15787=CARTESIAN_POINT('',(45.2458348754007,-78.3680848350663,-10.));
#15788=CARTESIAN_POINT('',(190.,13.,-10.));
#15789=CARTESIAN_POINT('Origin',(157.,-13.,9.));
#15790=CARTESIAN_POINT('Origin',(157.,13.,9.));
#15791=CARTESIAN_POINT('Origin',(184.75,0.,4.6));
#15792=CARTESIAN_POINT('Origin',(164.75,0.,4.6));
#15793=CARTESIAN_POINT('Origin',(195.2,-6.23205080756882,3.));
#15794=CARTESIAN_POINT('',(195.2,-6.23205080756882,3.));
#15795=CARTESIAN_POINT('',(195.2,-6.23205080756882,3.));
#15796=CARTESIAN_POINT('',(198.2,-7.9641016151377,3.));
#15797=CARTESIAN_POINT('',(195.2,-6.23205080756882,3.));
#15798=CARTESIAN_POINT('',(198.2,-7.9641016151377,3.));
#15799=CARTESIAN_POINT('Origin',(198.2,-7.9641016151377,3.));
#15800=CARTESIAN_POINT('',(201.2,-6.23205080756883,3.));
#15801=CARTESIAN_POINT('',(198.2,-7.9641016151377,3.));
#15802=CARTESIAN_POINT('',(201.2,-6.23205080756883,3.));
#15803=CARTESIAN_POINT('Origin',(201.2,-6.23205080756883,3.));
#15804=CARTESIAN_POINT('',(201.2,-2.76794919243107,3.));
#15805=CARTESIAN_POINT('',(201.2,-6.23205080756883,3.));
#15806=CARTESIAN_POINT('',(201.2,-2.76794919243107,3.));
#15807=CARTESIAN_POINT('Origin',(201.2,-2.76794919243107,3.));
#15808=CARTESIAN_POINT('',(198.2,-1.03589838486218,3.));
#15809=CARTESIAN_POINT('',(201.2,-2.76794919243107,3.));
#15810=CARTESIAN_POINT('',(198.2,-1.03589838486218,3.));
#15811=CARTESIAN_POINT('Origin',(198.2,-1.03589838486218,3.));
#15812=CARTESIAN_POINT('',(195.2,-2.76794919243105,3.));
#15813=CARTESIAN_POINT('',(198.2,-1.03589838486218,3.));
#15814=CARTESIAN_POINT('',(195.2,-2.76794919243105,3.));
#15815=CARTESIAN_POINT('Origin',(195.2,-2.76794919243105,3.));
#15816=CARTESIAN_POINT('',(195.2,-2.76794919243105,3.));
#15817=CARTESIAN_POINT('Origin',(0.,0.,3.));
#15818=CARTESIAN_POINT('Origin',(198.2,12.9641016151378,3.));
#15819=CARTESIAN_POINT('',(201.2,11.2320508075689,3.));
#15820=CARTESIAN_POINT('',(201.2,11.2320508075689,3.));
#15821=CARTESIAN_POINT('',(198.2,12.9641016151378,3.));
#15822=CARTESIAN_POINT('',(198.2,12.9641016151378,3.));
#15823=CARTESIAN_POINT('',(198.2,12.9641016151378,3.));
#15824=CARTESIAN_POINT('Origin',(195.2,11.2320508075689,3.));
#15825=CARTESIAN_POINT('',(195.2,11.2320508075689,3.));
#15826=CARTESIAN_POINT('',(195.2,11.2320508075689,3.));
#15827=CARTESIAN_POINT('',(195.2,11.2320508075689,3.));
#15828=CARTESIAN_POINT('Origin',(195.2,7.76794919243112,3.));
#15829=CARTESIAN_POINT('',(195.2,7.76794919243112,3.));
#15830=CARTESIAN_POINT('',(195.2,7.76794919243112,3.));
#15831=CARTESIAN_POINT('',(195.2,7.76794919243112,3.));
#15832=CARTESIAN_POINT('Origin',(198.2,6.03589838486225,3.));
#15833=CARTESIAN_POINT('',(198.2,6.03589838486225,3.));
#15834=CARTESIAN_POINT('',(198.2,6.03589838486225,3.));
#15835=CARTESIAN_POINT('',(198.2,6.03589838486225,3.));
#15836=CARTESIAN_POINT('Origin',(201.2,7.76794919243114,3.));
#15837=CARTESIAN_POINT('',(201.2,7.76794919243114,3.));
#15838=CARTESIAN_POINT('',(201.2,7.76794919243114,3.));
#15839=CARTESIAN_POINT('',(201.2,7.76794919243114,3.));
#15840=CARTESIAN_POINT('Origin',(201.2,11.2320508075689,3.));
#15841=CARTESIAN_POINT('',(201.2,11.2320508075689,3.));
#15842=CARTESIAN_POINT('Origin',(0.,0.,3.));
#15843=CARTESIAN_POINT('Origin',(0.,13.,0.));
#15844=CARTESIAN_POINT('',(203.5,13.,0.));
#15845=CARTESIAN_POINT('Origin',(205.,13.,0.));
#15846=CARTESIAN_POINT('',(205.,13.8660254037845,0.));
#15847=CARTESIAN_POINT('Origin',(205.,13.8660254037845,0.));
#15848=CARTESIAN_POINT('Origin',(0.,9.80814117218957E-17,1.));
#15849=CARTESIAN_POINT('',(155.,-3.95,1.));
#15850=CARTESIAN_POINT('',(155.,3.95,1.));
#15851=CARTESIAN_POINT('Origin',(155.,-3.95,1.));
#15852=CARTESIAN_POINT('Origin',(155.,3.95,1.));
#18833=UNCERTAINTY_MEASURE_WITH_UNIT(LENGTH_MEASURE(0.01),#18868,
'DISTANCE_ACCURACY_VALUE',
'Maximum model space distance between geometric entities at asserted c
onnectivities');
#18849=UNCERTAINTY_MEASURE_WITH_UNIT(LENGTH_MEASURE(0.01),#18868,
'DISTANCE_ACCURACY_VALUE',
'Maximum model space distance between geometric entities at asserted c
onnectivities');
#18851=(
GEOMETRIC_REPRESENTATION_CONTEXT(3)
GLOBAL_UNCERTAINTY_ASSIGNED_CONTEXT((#18833))
GLOBAL_UNIT_ASSIGNED_CONTEXT((#18868,#18870,#18871))
REPRESENTATION_CONTEXT('','3D')
);
#18867=(
GEOMETRIC_REPRESENTATION_CONTEXT(3)
GLOBAL_UNCERTAINTY_ASSIGNED_CONTEXT((#18849))
GLOBAL_UNIT_ASSIGNED_CONTEXT((#18868,#18870,#18871))
REPRESENTATION_CONTEXT('','3D')
);
#18868=(
LENGTH_UNIT()
NAMED_UNIT(*)
SI_UNIT(.MILLI.,.METRE.)
);
#18870=(
NAMED_UNIT(*)
PLANE_ANGLE_UNIT()
SI_UNIT($,.RADIAN.)
);
#18871=(
NAMED_UNIT(*)
SI_UNIT($,.STERADIAN.)
SOLID_ANGLE_UNIT()
);
#18873=SHAPE_DEFINITION_REPRESENTATION(#18890,#18935);
#18890=PRODUCT_DEFINITION_SHAPE('',$,#18953);
#18935=SHAPE_REPRESENTATION('',(#11160),#18851);
#18951=PRODUCT_DEFINITION_CONTEXT('part definition',#19004,'design');
#18953=PRODUCT_DEFINITION('Drive End Bracket 1','Drive End Bracket 1',#18970,
#18951);
#18970=PRODUCT_DEFINITION_FORMATION('',$,#19007);
#19004=APPLICATION_CONTEXT(
'Core Data for Automotive Mechanical Design Process');
#19005=PRODUCT_CONTEXT('part definition',#19004,'mechanical');
#19007=PRODUCT('Drive End Bracket 1','Drive End Bracket 1',$,(#19005));
#19024=PRESENTATION_STYLE_ASSIGNMENT((#19030));
#19030=SURFACE_STYLE_USAGE(.BOTH.,#19036);
#19036=SURFACE_SIDE_STYLE('',(#19042));
#19042=SURFACE_STYLE_FILL_AREA(#19048);
#19048=FILL_AREA_STYLE('Opaque(20,51,87)',(#19054));
#19054=FILL_AREA_STYLE_COLOUR('Opaque(20,51,87)',#19060);
#19060=COLOUR_RGB('Opaque(20,51,87)',0.0784313725490196,0.2,0.341176470588235);
ENDSEC;
END-ISO-10303-21;
